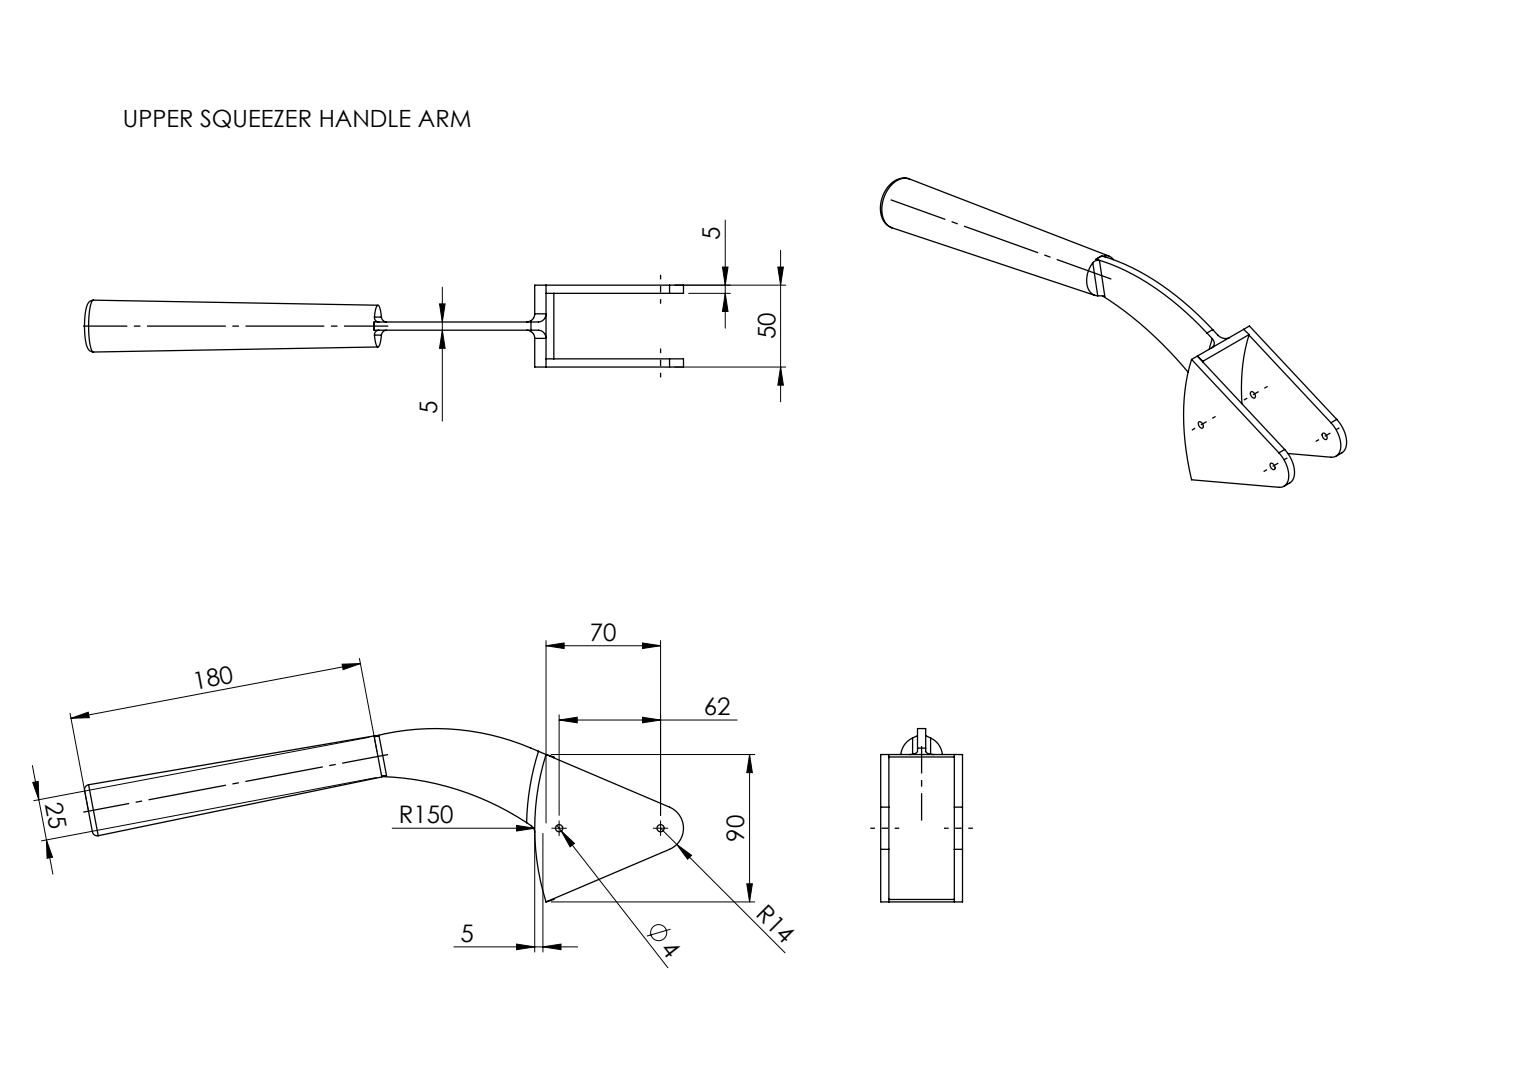
ISO-10303-21;
HEADER;
FILE_DESCRIPTION (('STEP AP214'),
    '1' );
FILE_NAME ('Upper Squeezer Handle Arm.step',
    '2026-10-02T13:02:33',
    ( '' ),
    ( '' ),
    'SwSTEP 2.0',
    'SolidWorks 2026',
    '' );
FILE_SCHEMA (( 'AUTOMOTIVE_DESIGN' ));
ENDSEC;

DATA;
#40=ORIENTED_EDGE ( 'NONE', *, *, #10473, .T. ) ;
#56=VERTEX_POINT ( 'NONE', #8559 ) ;
#88=DIRECTION ( 'NONE',  ( -0.000000000000000000, -0.000000000000000000, -1.000000000000000000 ) ) ;
#109=( NAMED_UNIT ( * ) SI_UNIT ( $, .STERADIAN. ) SOLID_ANGLE_UNIT ( ) );
#113=VERTEX_POINT ( 'NONE', #1359 ) ;
#130=FACE_OUTER_BOUND ( 'NONE', #4986, .T. ) ;
#141=DIRECTION ( 'NONE',  ( -1.000000000000000000, 0.000000000000000000, 0.000000000000000000 ) ) ;
#142=EDGE_LOOP ( 'NONE', ( #9264, #8766, #6960, #18741, #15276 ) ) ;
#165=CIRCLE ( 'NONE', #14403, 12.74754878398197633 ) ;
#196=CARTESIAN_POINT ( 'NONE',  ( -64.20000000000000284, 2.694222958124180951E-16, -25.00000000000000000 ) ) ;
#229=ORIENTED_EDGE ( 'NONE', *, *, #5595, .F. ) ;
#256=DIRECTION ( 'NONE',  ( 0.000000000000000000, 0.000000000000000000, 1.000000000000000000 ) ) ;
#276=ORIENTED_EDGE ( 'NONE', *, *, #13888, .T. ) ;
#288=DIRECTION ( 'NONE',  ( 0.9826218788918642533, 0.1856185419698762884, -0.000000000000000000 ) ) ;
#289=AXIS2_PLACEMENT_3D ( 'NONE', #791, #6676, #10995 ) ;
#326=ORIENTED_EDGE ( 'NONE', *, *, #13082, .F. ) ;
#359=EDGE_CURVE ( 'NONE', #9050, #9141, #4270, .T. ) ;
#361=DIRECTION ( 'NONE',  ( 0.000000000000000000, 0.000000000000000000, 1.000000000000000000 ) ) ;
#395=LINE ( 'NONE', #17952, #3848 ) ;
#411=VERTEX_POINT ( 'NONE', #18575 ) ;
#417=DIRECTION ( 'NONE',  ( 1.000000000000000000, 0.000000000000000000, 0.000000000000000000 ) ) ;
#426=TOROIDAL_SURFACE ( 'NONE', #13412, 155.0000000000000284, 5.000000000000000000 ) ;
#430=CARTESIAN_POINT ( 'NONE',  ( -349.0394899966146909, 23.59157312255261729, 2.567204941047426911E-15 ) ) ;
#468=LINE ( 'NONE', #1619, #12903 ) ;
#479=DIRECTION ( 'NONE',  ( -1.000000000000000000, 0.000000000000000000, 0.000000000000000000 ) ) ;
#496=CARTESIAN_POINT ( 'NONE',  ( -174.0670050711101737, 56.28339404658832024, -2.500000000000000000 ) ) ;
#512=CARTESIAN_POINT ( 'NONE',  ( 5.481473465377026066, -12.88229205725314586, -19.99999999999999645 ) ) ;
#518=VERTEX_POINT ( 'NONE', #6943 ) ;
#522=DIRECTION ( 'NONE',  ( -0.000000000000000000, -0.000000000000000000, -1.000000000000000000 ) ) ;
#530=FACE_BOUND ( 'NONE', #4136, .T. ) ;
#536=FACE_OUTER_BOUND ( 'NONE', #6098, .T. ) ;
#552=ADVANCED_FACE ( 'NONE', ( #6251 ), #11983, .T. ) ;
#558=LINE ( 'NONE', #16393, #11124 ) ;
#559=VECTOR ( 'NONE', #18084, 1000.000000000000000 ) ;
#563=FACE_OUTER_BOUND ( 'NONE', #9796, .T. ) ;
#564=EDGE_CURVE ( 'NONE', #10544, #13205, #12684, .T. ) ;
#574=CARTESIAN_POINT ( 'NONE',  ( -2.200000000000000178, 0.000000000000000000, 25.00000000000000000 ) ) ;
#575=CIRCLE ( 'NONE', #15701, 2.200000000000000622 ) ;
#607=VECTOR ( 'NONE', #8603, 1000.000000000000000 ) ;
#619=ORIENTED_EDGE ( 'NONE', *, *, #10277, .T. ) ;
#671=PLANE ( 'NONE',  #9426 ) ;
#679=CARTESIAN_POINT ( 'NONE',  ( -70.00000000000000000, 44.99999999999999289, -19.99999999999999645 ) ) ;
#718=CARTESIAN_POINT ( 'NONE',  ( -174.0586467429681363, 56.10169251196822415, -3.278196957010492962 ) ) ;
#742=DIRECTION ( 'NONE',  ( 0.000000000000000000, 0.000000000000000000, 1.000000000000000000 ) ) ;
#744=( LENGTH_UNIT ( ) NAMED_UNIT ( * ) SI_UNIT ( .MILLI., .METRE. ) );
#748=LINE ( 'NONE', #7752, #16988 ) ;
#751=DIRECTION ( 'NONE',  ( 1.000000000000000000, 0.000000000000000000, 0.000000000000000000 ) ) ;
#753=VERTEX_POINT ( 'NONE', #12822 ) ;
#780=CARTESIAN_POINT ( 'NONE',  ( 73.09088021254186174, 1.387778780781445676E-14, 25.00000000000000000 ) ) ;
#783=EDGE_CURVE ( 'NONE', #1828, #11020, #12691, .T. ) ;
#791=CARTESIAN_POINT ( 'NONE',  ( -70.00000000000000000, 44.99999999999999289, 2.500000000000000000 ) ) ;
#797=ORIENTED_EDGE ( 'NONE', *, *, #18408, .F. ) ;
#830=CIRCLE ( 'NONE', #16252, 2.200000000000007283 ) ;
#836=CARTESIAN_POINT ( 'NONE',  ( -346.6567719130321166, 10.97801148527007697, 9.951701414186830458E-16 ) ) ;
#844=DIRECTION ( 'NONE',  ( -0.000000000000000000, -0.000000000000000000, -1.000000000000000000 ) ) ;
#860=AXIS2_PLACEMENT_3D ( 'NONE', #11980, #10856, #3558 ) ;
#883=VECTOR ( 'NONE', #7257, 1000.000000000000000 ) ;
#897=VERTEX_POINT ( 'NONE', #15494 ) ;
#901=CARTESIAN_POINT ( 'NONE',  ( -168.2745196454702068, 32.00972194781247282, -2.584671478510871090 ) ) ;
#912=VECTOR ( 'NONE', #7964, 1000.000000000000000 ) ;
#918=CIRCLE ( 'NONE', #5451, 150.0000000000000284 ) ;
#955=EDGE_CURVE ( 'NONE', #4610, #5412, #8486, .T. ) ;
#985=EDGE_LOOP ( 'NONE', ( #11976, #13924 ) ) ;
#987=VECTOR ( 'NONE', #3572, 1000.000000000000000 ) ;
#997=CARTESIAN_POINT ( 'NONE',  ( 73.09088021254186174, 1.387778780781445676E-14, 7.500000000000000000 ) ) ;
#998=CARTESIAN_POINT ( 'NONE',  ( 73.09088021254186174, 1.387778780781445676E-14, -7.500000000000000000 ) ) ;
#1008=ORIENTED_EDGE ( 'NONE', *, *, #2884, .T. ) ;
#1058=CARTESIAN_POINT ( 'NONE',  ( 2.200000000000000178, 2.694222958124177006E-16, 25.00000000000000000 ) ) ;
#1064=CARTESIAN_POINT ( 'NONE',  ( -167.4745151998187680, 32.15905408292213252, 2.500000000000000000 ) ) ;
#1084=CARTESIAN_POINT ( 'NONE',  ( -170.4124675745486570, 31.54971992778986234, -5.500000000000000000 ) ) ;
#1099=CARTESIAN_POINT ( 'NONE',  ( -170.5500158571522320, 32.36820283781686669, 5.132104245558541500 ) ) ;
#1103=CARTESIAN_POINT ( 'NONE',  ( -70.00000000000000000, 44.99999999999999289, 7.500000000000007105 ) ) ;
#1128=CARTESIAN_POINT ( 'NONE',  ( 0.000000000000000000, 0.000000000000000000, 25.00000000000000000 ) ) ;
#1130=CARTESIAN_POINT ( 'NONE',  ( -65.23030399291528170, -43.49999999999991473, 19.99999999999993605 ) ) ;
#1144=ORIENTED_EDGE ( 'NONE', *, *, #12791, .F. ) ;
#1151=DIRECTION ( 'NONE',  ( -0.9826218788918642533, -0.1856185419698762884, 0.000000000000000000 ) ) ;
#1160=DIRECTION ( 'NONE',  ( 1.000000000000000000, 0.000000000000000000, 0.000000000000000000 ) ) ;
#1162=CIRCLE ( 'NONE', #11700, 145.0000000000000284 ) ;
#1165=DIRECTION ( 'NONE',  ( -0.000000000000000000, -0.000000000000000000, 1.000000000000000000 ) ) ;
#1181=LINE ( 'NONE', #16691, #8739 ) ;
#1194=FACE_OUTER_BOUND ( 'NONE', #3187, .T. ) ;
#1215=LINE ( 'NONE', #7000, #4553 ) ;
#1220=ADVANCED_FACE ( 'NONE', ( #9641 ), #2329, .T. ) ;
#1222=LINE ( 'NONE', #12750, #18237 ) ;
#1227=CIRCLE ( 'NONE', #16352, 12.74754878398197633 ) ;
#1235=CARTESIAN_POINT ( 'NONE',  ( -70.00000000000000000, 44.99999999999999289, 20.00000000000001776 ) ) ;
#1238=AXIS2_PLACEMENT_3D ( 'NONE', #16759, #16849, #17042 ) ;
#1258=ORIENTED_EDGE ( 'NONE', *, *, #6088, .F. ) ;
#1262=CARTESIAN_POINT ( 'NONE',  ( -170.4124675745486570, 31.54971992778987655, 2.500000000000000000 ) ) ;
#1280=CARTESIAN_POINT ( 'NONE',  ( -344.2740538294495423, -1.635550152012466452, 9.951701414186830458E-16 ) ) ;
#1299=CARTESIAN_POINT ( 'NONE',  ( -174.8673125818257006, 55.13264502119463373, 5.500000000000001776 ) ) ;
#1331=EDGE_CURVE ( 'NONE', #7954, #16292, #18686, .T. ) ;
#1337=CARTESIAN_POINT ( 'NONE',  ( 73.09088021254186174, 1.387778780781445676E-14, 19.99999999999997513 ) ) ;
#1339=DIRECTION ( 'NONE',  ( -0.3915338189555019333, 0.9201637183752250371, 0.000000000000000000 ) ) ;
#1344=PLANE ( 'NONE',  #13494 ) ;
#1359=CARTESIAN_POINT ( 'NONE',  ( -2.200000000000000178, 0.000000000000000000, -19.99999999999999645 ) ) ;
#1393=CARTESIAN_POINT ( 'NONE',  ( -175.0529311237955596, 56.11526690008648899, 2.500000000000000000 ) ) ;
#1405=FACE_OUTER_BOUND ( 'NONE', #1455, .T. ) ;
#1409=CARTESIAN_POINT ( 'NONE',  ( -170.4124675745486570, 31.54971992778987655, -2.500000000000000000 ) ) ;
#1410=ORIENTED_EDGE ( 'NONE', *, *, #11519, .F. ) ;
#1417=EDGE_CURVE ( 'NONE', #1906, #5889, #1222, .T. ) ;
#1455=EDGE_LOOP ( 'NONE', ( #13094, #13490 ) ) ;
#1475=CARTESIAN_POINT ( 'NONE',  ( -70.24339520416560845, 45.10356575889633746, -5.890567936347699707 ) ) ;
#1513=AXIS2_PLACEMENT_3D ( 'NONE', #9646, #10955, #3741 ) ;
#1515=DIRECTION ( 'NONE',  ( -2.671473304378624222E-16, -0.000000000000000000, -1.000000000000000000 ) ) ;
#1526=EDGE_LOOP ( 'NONE', ( #6897, #6518, #14749, #5534 ) ) ;
#1527=ADVANCED_FACE ( 'NONE', ( #13477 ), #6129, .T. ) ;
#1539=CARTESIAN_POINT ( 'NONE',  ( -76.95187462163347902, -1.796833398359349410, -6.747090334426651737 ) ) ;
#1549=DIRECTION ( 'NONE',  ( -0.000000000000000000, -0.000000000000000000, -1.000000000000000000 ) ) ;
#1566=AXIS2_PLACEMENT_3D ( 'NONE', #9927, #1151, #9845 ) ;
#1571=CARTESIAN_POINT ( 'NONE',  ( -76.90911978745816668, -45.00000000000000711, 20.00000000000002132 ) ) ;
#1600=ORIENTED_EDGE ( 'NONE', *, *, #16700, .T. ) ;
#1615=LINE ( 'NONE', #17277, #8663 ) ;
#1619=CARTESIAN_POINT ( 'NONE',  ( -69.99999999999998579, -45.00000000000000711, -19.99999999999999645 ) ) ;
#1624=ORIENTED_EDGE ( 'NONE', *, *, #11579, .F. ) ;
#1629=CARTESIAN_POINT ( 'NONE',  ( -77.83221577883584530, 0.3113175352389498385, -4.597871329320426526 ) ) ;
#1646=DIRECTION ( 'NONE',  ( -0.3000000000000013767, -0.9539392014169453260, 0.000000000000000000 ) ) ;
#1679=AXIS2_PLACEMENT_3D ( 'NONE', #1950, #4958, #16653 ) ;
#1681=CARTESIAN_POINT ( 'NONE',  ( 73.09088021254186174, 1.387778780781445676E-14, -2.500000000000000444 ) ) ;
#1706=AXIS2_PLACEMENT_3D ( 'NONE', #9851, #15620, #2647 ) ;
#1719=ORIENTED_EDGE ( 'NONE', *, *, #16557, .T. ) ;
#1720=ORIENTED_EDGE ( 'NONE', *, *, #1770, .F. ) ;
#1732=DIRECTION ( 'NONE',  ( -0.000000000000000000, -0.000000000000000000, 1.000000000000000000 ) ) ;
#1734=CARTESIAN_POINT ( 'NONE',  ( -70.46959788260221558, 45.19981602042874869, -5.279908564046689179 ) ) ;
#1770=EDGE_CURVE ( 'NONE', #11020, #1828, #4868, .T. ) ;
#1780=VECTOR ( 'NONE', #11064, 1000.000000000000114 ) ;
#1828=VERTEX_POINT ( 'NONE', #15612 ) ;
#1846=FACE_OUTER_BOUND ( 'NONE', #15073, .T. ) ;
#1855=AXIS2_PLACEMENT_3D ( 'NONE', #430, #3432, #1939 ) ;
#1863=DIRECTION ( 'NONE',  ( 0.000000000000000000, 0.000000000000000000, 1.000000000000000000 ) ) ;
#1883=ORIENTED_EDGE ( 'NONE', *, *, #14085, .T. ) ;
#1906=VERTEX_POINT ( 'NONE', #3176 ) ;
#1916=CARTESIAN_POINT ( 'NONE',  ( 5.481473465377021625, 12.88229205725314763, -19.99999999999998934 ) ) ;
#1923=DIRECTION ( 'NONE',  ( 0.9201637183752249260, -0.3915338189555017667, 0.000000000000000000 ) ) ;
#1936=DIRECTION ( 'NONE',  ( -0.000000000000000000, -0.000000000000000000, -1.000000000000000000 ) ) ;
#1939=DIRECTION ( 'NONE',  ( 0.000000000000000000, -1.000000000000000000, -1.203364738757079611E-16 ) ) ;
#1950=CARTESIAN_POINT ( 'NONE',  ( -76.90911978745816668, -45.00000000000000711, 20.00000000000002132 ) ) ;
#1980=ORIENTED_EDGE ( 'NONE', *, *, #10414, .F. ) ;
#1995=CARTESIAN_POINT ( 'NONE',  ( 73.09088021254186174, 1.387778780781445676E-14, 19.99999999999997513 ) ) ;
#2005=EDGE_CURVE ( 'NONE', #8575, #3590, #2409, .T. ) ;
#2012=PLANE ( 'NONE',  #13053 ) ;
#2027=DIRECTION ( 'NONE',  ( 0.000000000000000000, 0.000000000000000000, 1.000000000000000000 ) ) ;
#2035=CARTESIAN_POINT ( 'NONE',  ( -172.7326993491721225, 43.83249341393818810, 9.951701414186830458E-16 ) ) ;
#2068=DIRECTION ( 'NONE',  ( -0.3915338189555018222, -0.9201637183752250371, 0.000000000000000000 ) ) ;
#2073=CARTESIAN_POINT ( 'NONE',  ( -172.7326993491721225, 43.83249341393818810, 9.951701414186830458E-16 ) ) ;
#2082=CYLINDRICAL_SURFACE ( 'NONE', #10230, 13.99999999999999822 ) ;
#2097=ORIENTED_EDGE ( 'NONE', *, *, #3220, .T. ) ;
#2113=CARTESIAN_POINT ( 'NONE',  ( -73.13054148225640461, 46.33205954274173877, -2.756412765970647882 ) ) ;
#2121=AXIS2_PLACEMENT_3D ( 'NONE', #8067, #6961, #11086 ) ;
#2122=AXIS2_PLACEMENT_3D ( 'NONE', #10418, #12980, #8826 ) ;
#2124=CARTESIAN_POINT ( 'NONE',  ( -169.3344985746950044, 31.92300743893811088, 3.146712427857110583 ) ) ;
#2127=TOROIDAL_SURFACE ( 'NONE', #16361, 155.0000000000000284, 5.000000000000000000 ) ;
#2132=CARTESIAN_POINT ( 'NONE',  ( -175.0529311237955596, 56.11526690008648899, 2.500000000000000000 ) ) ;
#2138=VERTEX_POINT ( 'NONE', #7622 ) ;
#2144=VERTEX_POINT ( 'NONE', #4755 ) ;
#2147=CIRCLE ( 'NONE', #13934, 2.200000000000000178 ) ;
#2153=DIRECTION ( 'NONE',  ( 1.000000000000000000, 0.000000000000000000, -0.000000000000000000 ) ) ;
#2156=DIRECTION ( 'NONE',  ( -1.000000000000000000, 0.000000000000000000, 0.000000000000000000 ) ) ;
#2167=DIRECTION ( 'NONE',  ( 0.000000000000000000, 0.000000000000000000, 1.000000000000000000 ) ) ;
#2172=ADVANCED_FACE ( 'NONE', ( #10535 ), #2012, .F. ) ;
#2174=AXIS2_PLACEMENT_3D ( 'NONE', #12078, #3652, #16476 ) ;
#2196=FILL_AREA_STYLE ('',( #9865 ) ) ;
#2201=DIRECTION ( 'NONE',  ( -0.9201637183752250371, 0.3915338189555017667, 2.458192809297184296E-16 ) ) ;
#2209=EDGE_CURVE ( 'NONE', #4027, #10083, #12700, .T. ) ;
#2212=ORIENTED_EDGE ( 'NONE', *, *, #9806, .T. ) ;
#2231=ORIENTED_EDGE ( 'NONE', *, *, #18528, .T. ) ;
#2232=CARTESIAN_POINT ( 'NONE',  ( -79.20163718375225415, 48.91533818955501545, 2.500000000000000000 ) ) ;
#2260=CARTESIAN_POINT ( 'NONE',  ( -80.88842949533930948, 2.743677230443736903, -2.574918967431987227 ) ) ;
#2268=DIRECTION ( 'NONE',  ( -0.9826218788918642533, -0.1856185419698762884, 0.000000000000000000 ) ) ;
#2276=FACE_BOUND ( 'NONE', #7402, .T. ) ;
#2285=FACE_OUTER_BOUND ( 'NONE', #5660, .T. ) ;
#2290=LINE ( 'NONE', #8071, #9863 ) ;
#2295=CARTESIAN_POINT ( 'NONE',  ( -169.9074338689577530, 31.96868808717145782, -3.724467847532850762 ) ) ;
#2305=CARTESIAN_POINT ( 'NONE',  ( -74.62210677719829732, 46.96672731380024146, 2.500000000000000000 ) ) ;
#2315=ORIENTED_EDGE ( 'NONE', *, *, #14957, .T. ) ;
#2329=PLANE ( 'NONE',  #12706 ) ;
#2359=CARTESIAN_POINT ( 'NONE',  ( -69.99999999999998579, -45.00000000000000711, 25.00000000000000000 ) ) ;
#2372=EDGE_CURVE ( 'NONE', #14394, #2138, #11538, .T. ) ;
#2389=CARTESIAN_POINT ( 'NONE',  ( -170.5980861165185445, 32.53234180668174247, -5.500000000000001776 ) ) ;
#2397=ORIENTED_EDGE ( 'NONE', *, *, #5880, .F. ) ;
#2408=CARTESIAN_POINT ( 'NONE',  ( -72.99658078354744362, 46.27505866028131010, 2.816616659167352044 ) ) ;
#2409=LINE ( 'NONE', #11012, #5208 ) ;
#2415=ORIENTED_EDGE ( 'NONE', *, *, #16291, .F. ) ;
#2441=DIRECTION ( 'NONE',  ( 0.1856185419698762884, -0.9826218788918642533, 0.000000000000000000 ) ) ;
#2446=DIRECTION ( 'NONE',  ( 0.000000000000000000, 0.000000000000000000, 1.000000000000000000 ) ) ;
#2453=LINE ( 'NONE', #1058, #9909 ) ;
#2465=CARTESIAN_POINT ( 'NONE',  ( -79.48103206242137730, 1.792378103397237687, -3.092380961970916609 ) ) ;
#2472=AXIS2_PLACEMENT_3D ( 'NONE', #5439, #3997, #13856 ) ;
#2481=FACE_BOUND ( 'NONE', #6430, .T. ) ;
#2508=CARTESIAN_POINT ( 'NONE',  ( -71.81027153490798298, 45.77027871590120611, 3.518396351564663682 ) ) ;
#2530=CARTESIAN_POINT ( 'NONE',  ( -167.4745151998187680, 32.15905408292206147, -2.500000000000000000 ) ) ;
#2557=CYLINDRICAL_SURFACE ( 'NONE', #16277, 2.200000000000000622 ) ;
#2572=ORIENTED_EDGE ( 'NONE', *, *, #16811, .F. ) ;
#2574=ADVANCED_FACE ( 'NONE', ( #8157 ), #8849, .T. ) ;
#2575=ORIENTED_EDGE ( 'NONE', *, *, #4514, .T. ) ;
#2594=VECTOR ( 'NONE', #13746, 1000.000000000000000 ) ;
#2595=CARTESIAN_POINT ( 'NONE',  ( -70.03008040050728766, 45.01279934630233015, 6.841710791646147705 ) ) ;
#2597=CARTESIAN_POINT ( 'NONE',  ( 0.000000000000000000, 0.000000000000000000, -19.99999999999999645 ) ) ;
#2626=CARTESIAN_POINT ( 'NONE',  ( -76.94165664733894516, -1.794943808410583763, 6.745229976240270098 ) ) ;
#2647=DIRECTION ( 'NONE',  ( -1.000000000000000000, 0.000000000000000000, 0.000000000000000000 ) ) ;
#2660=EDGE_CURVE ( 'NONE', #18388, #3138, #17169, .T. ) ;
#2664=AXIS2_PLACEMENT_3D ( 'NONE', #4048, #15343, #8340 ) ;
#2687=ADVANCED_FACE ( 'NONE', ( #15728 ), #2557, .F. ) ;
#2691=ADVANCED_FACE ( 'NONE', ( #17279, #6940, #5509 ), #1344, .F. ) ;
#2731=B_SPLINE_CURVE_WITH_KNOTS ( 'NONE', 3,
 ( #15742, #17379, #4363, #12879 ),
 .UNSPECIFIED., .F., .F.,
 ( 4, 4 ),
 ( 0.000000000000000000, 0.003000475340473851647 ),
 .UNSPECIFIED. ) ;
#2740=CARTESIAN_POINT ( 'NONE',  ( -168.4538323585589694, 31.95594125380575434, 2.500000000000000000 ) ) ;
#2744=PLANE ( 'NONE',  #4472 ) ;
#2764=EDGE_LOOP ( 'NONE', ( #5604, #4078, #18302, #15584 ) ) ;
#2770=CARTESIAN_POINT ( 'NONE',  ( -77.50987606495345972, -0.1965428547086033040, -5.115516238835398966 ) ) ;
#2787=B_SPLINE_CURVE_WITH_KNOTS ( 'NONE', 3,
 ( #2389, #15281, #16923, #13956, #12524, #10912, #15377, #2295, #6578, #18367, #12327, #13849, #16736, #901, #12436, #5340 ),
 .UNSPECIFIED., .F., .F.,
 ( 4, 2, 2, 2, 2, 2, 2, 4 ),
 ( 1.734723475976807094E-18, 0.0006035471611761681829, 0.001207094322352334631, 0.001810641483528501296, 0.002414188644704666660, 0.003017735805880831807, 0.003621282967056997388, 0.004828377289409254390 ),
 .UNSPECIFIED. ) ;
#2827=ORIENTED_EDGE ( 'NONE', *, *, #2372, .T. ) ;
#2853=DIRECTION ( 'NONE',  ( -0.1856185419698762884, 0.9826218788918642533, 0.000000000000000000 ) ) ;
#2859=DIRECTION ( 'NONE',  ( 1.000000000000000000, 0.000000000000000000, 0.000000000000000000 ) ) ;
#2868=CARTESIAN_POINT ( 'NONE',  ( -172.8945038000772456, 56.46685571404672999, 2.584671478510881748 ) ) ;
#2872=CARTESIAN_POINT ( 'NONE',  ( -70.03007184274690644, 45.01279570493660742, -6.843761338458851817 ) ) ;
#2884=EDGE_CURVE ( 'NONE', #12460, #518, #18423, .T. ) ;
#2899=ORIENTED_EDGE ( 'NONE', *, *, #11873, .T. ) ;
#2903=EDGE_CURVE ( 'NONE', #14167, #1906, #558, .T. ) ;
#2923=ORIENTED_EDGE ( 'NONE', *, *, #17865, .F. ) ;
#2927=CIRCLE ( 'NONE', #13510, 155.0000000000000284 ) ;
#2931=DIRECTION ( 'NONE',  ( 1.000000000000000000, 0.000000000000000000, -0.000000000000000000 ) ) ;
#2954=EDGE_LOOP ( 'NONE', ( #14575, #6574, #14958, #16245 ) ) ;
#2964=ORIENTED_EDGE ( 'NONE', *, *, #17775, .T. ) ;
#2966=CARTESIAN_POINT ( 'NONE',  ( 0.000000000000000000, 0.000000000000000000, 25.00000000000000000 ) ) ;
#2970=AXIS2_PLACEMENT_3D ( 'NONE', #2966, #4104, #141 ) ;
#2986=PLANE ( 'NONE',  #12549 ) ;
#3010=LINE ( 'NONE', #12955, #8538 ) ;
#3012=DIRECTION ( 'NONE',  ( 1.000000000000000000, 0.000000000000000000, 0.000000000000000000 ) ) ;
#3014=CARTESIAN_POINT ( 'NONE',  ( 0.000000000000000000, 0.000000000000000000, 20.00000000000000000 ) ) ;
#3037=CIRCLE ( 'NONE', #9719, 171.3327290851023292 ) ;
#3062=EDGE_LOOP ( 'NONE', ( #8219, #13627 ) ) ;
#3066=CARTESIAN_POINT ( 'NONE',  ( -174.8824303167912717, 55.30300876447670788, -5.132104245558540612 ) ) ;
#3067=CARTESIAN_POINT ( 'NONE',  ( -71.14323843904776368, 45.48645312032893173, -4.192014029982320977 ) ) ;
#3069=ORIENTED_EDGE ( 'NONE', *, *, #16811, .T. ) ;
#3083=DIRECTION ( 'NONE',  ( -0.000000000000000000, -0.000000000000000000, -1.000000000000000000 ) ) ;
#3087=ORIENTED_EDGE ( 'NONE', *, *, #4173, .F. ) ;
#3123=EDGE_CURVE ( 'NONE', #753, #7914, #8693, .T. ) ;
#3138=VERTEX_POINT ( 'NONE', #17523 ) ;
#3147=DIRECTION ( 'NONE',  ( 1.000000000000000000, 0.000000000000000000, 0.000000000000000000 ) ) ;
#3148=DIRECTION ( 'NONE',  ( 0.9201637183752249260, 0.3915338189555018777, -2.458192809297183803E-16 ) ) ;
#3176=CARTESIAN_POINT ( 'NONE',  ( -69.99999999999998579, -45.00000000000000711, 20.00000000000001776 ) ) ;
#3187=EDGE_LOOP ( 'NONE', ( #7835, #12831, #11103, #4991, #2315, #2899 ) ) ;
#3197=DIRECTION ( 'NONE',  ( 0.1856185419698760941, -0.9826218788918640312, 0.000000000000000000 ) ) ;
#3204=ORIENTED_EDGE ( 'NONE', *, *, #4750, .F. ) ;
#3209=ORIENTED_EDGE ( 'NONE', *, *, #18358, .F. ) ;
#3220=EDGE_CURVE ( 'NONE', #12815, #17451, #5025, .T. ) ;
#3230=VERTEX_POINT ( 'NONE', #15890 ) ;
#3249=DIRECTION ( 'NONE',  ( 1.000000000000000000, 0.000000000000000000, -2.671473304378624222E-16 ) ) ;
#3284=ORIENTED_EDGE ( 'NONE', *, *, #4389, .T. ) ;
#3293=VECTOR ( 'NONE', #7540, 1000.000000000000000 ) ;
#3295=CARTESIAN_POINT ( 'NONE',  ( -76.88766983611584749, -2.536636612185957595, -7.500000000000000000 ) ) ;
#3309=DIRECTION ( 'NONE',  ( 0.9201637183752249260, 0.3915338189555018777, 0.000000000000000000 ) ) ;
#3314=CARTESIAN_POINT ( 'NONE',  ( -59.79999999999999716, 0.000000000000000000, -25.00000000000000000 ) ) ;
#3326=CARTESIAN_POINT ( 'NONE',  ( -70.00000000000000000, 44.99999999999999289, 25.00000000000000000 ) ) ;
#3332=FACE_OUTER_BOUND ( 'NONE', #1526, .T. ) ;
#3362=ORIENTED_EDGE ( 'NONE', *, *, #18484, .T. ) ;
#3390=PRODUCT_DEFINITION_CONTEXT ( 'detailed design', #12682, 'design' ) ;
#3400=DIRECTION ( 'NONE',  ( -0.000000000000000000, -0.000000000000000000, -1.000000000000000000 ) ) ;
#3413=TOROIDAL_SURFACE ( 'NONE', #5868, 12.83663829214476770, 3.000000000000000000 ) ;
#3429=DIRECTION ( 'NONE',  ( -0.9826218788918641422, -0.1856185419698762606, 0.000000000000000000 ) ) ;
#3432=DIRECTION ( 'NONE',  ( 2.273171532858076093E-17, -1.203364738757079611E-16, 1.000000000000000000 ) ) ;
#3438=DIRECTION ( 'NONE',  ( -0.9826218788918642533, -0.1856185419698762884, 0.000000000000000000 ) ) ;
#3439=CARTESIAN_POINT ( 'NONE',  ( 73.09088021254186174, 1.387778780781445676E-14, -19.99999999999999645 ) ) ;
#3456=CYLINDRICAL_SURFACE ( 'NONE', #10978, 150.0000000000000284 ) ;
#3457=CARTESIAN_POINT ( 'NONE',  ( -172.7326993491721225, 43.83249341393818810, 9.951701414186830458E-16 ) ) ;
#3492=ORIENTED_EDGE ( 'NONE', *, *, #7729, .F. ) ;
#3496=ORIENTED_EDGE ( 'NONE', *, *, #6088, .T. ) ;
#3513=DIRECTION ( 'NONE',  ( 0.000000000000000000, 0.000000000000000000, 1.000000000000000000 ) ) ;
#3517=ORIENTED_EDGE ( 'NONE', *, *, #8216, .T. ) ;
#3530=DIRECTION ( 'NONE',  ( -0.000000000000000000, -0.000000000000000000, -1.000000000000000000 ) ) ;
#3537=ORIENTED_EDGE ( 'NONE', *, *, #18192, .T. ) ;
#3543=EDGE_LOOP ( 'NONE', ( #7602, #3069 ) ) ;
#3558=DIRECTION ( 'NONE',  ( 1.000000000000000000, 0.000000000000000000, 0.000000000000000000 ) ) ;
#3561=EDGE_CURVE ( 'NONE', #10291, #16721, #11039, .T. ) ;
#3572=DIRECTION ( 'NONE',  ( -0.000000000000000000, -0.000000000000000000, -1.000000000000000000 ) ) ;
#3573=UNCERTAINTY_MEASURE_WITH_UNIT (LENGTH_MEASURE( 1.000000000000000082E-05 ), #744, 'distance_accuracy_value', 'NONE');
#3581=EDGE_CURVE ( 'NONE', #16919, #13271, #5387, .T. ) ;
#3590=VERTEX_POINT ( 'NONE', #1235 ) ;
#3593=CARTESIAN_POINT ( 'NONE',  ( 2.200000000000000178, 2.694222958124177006E-16, -25.00000000000000000 ) ) ;
#3614=LINE ( 'NONE', #12527, #11561 ) ;
#3622=LINE ( 'NONE', #9430, #3293 ) ;
#3637=ORIENTED_EDGE ( 'NONE', *, *, #4750, .T. ) ;
#3644=ORIENTED_EDGE ( 'NONE', *, *, #3220, .F. ) ;
#3652=DIRECTION ( 'NONE',  ( 0.000000000000000000, 0.000000000000000000, 1.000000000000000000 ) ) ;
#3662=AXIS2_PLACEMENT_3D ( 'NONE', #12821, #5908, #17400 ) ;
#3663=CARTESIAN_POINT ( 'NONE',  ( -69.99999999999998579, -45.00000000000000711, 25.00000000000000000 ) ) ;
#3669=DIRECTION ( 'NONE',  ( -0.9826218788918641422, -0.1856185419698762606, 0.000000000000000000 ) ) ;
#3674=DIRECTION ( 'NONE',  ( -0.3915338189555019333, 0.9201637183752250371, 0.000000000000000000 ) ) ;
#3687=ORIENTED_EDGE ( 'NONE', *, *, #4439, .F. ) ;
#3690=PLANE ( 'NONE',  #13481 ) ;
#3695=ORIENTED_EDGE ( 'NONE', *, *, #7288, .F. ) ;
#3697=AXIS2_PLACEMENT_3D ( 'NONE', #8454, #13163, #2931 ) ;
#3702=DIRECTION ( 'NONE',  ( 1.000000000000000000, 0.000000000000000000, 0.000000000000000000 ) ) ;
#3705=VERTEX_POINT ( 'NONE', #9314 ) ;
#3707=DIRECTION ( 'NONE',  ( 3.816390434826605238E-17, 0.000000000000000000, -1.000000000000000000 ) ) ;
#3741=DIRECTION ( 'NONE',  ( 1.000000000000000000, 0.000000000000000000, 0.000000000000000000 ) ) ;
#3757=ORIENTED_EDGE ( 'NONE', *, *, #4389, .F. ) ;
#3758=CARTESIAN_POINT ( 'NONE',  ( -2.200000000000000178, 0.000000000000000000, -25.00000000000000000 ) ) ;
#3775=VERTEX_POINT ( 'NONE', #14690 ) ;
#3787=EDGE_CURVE ( 'NONE', #4836, #16919, #17591, .T. ) ;
#3842=ORIENTED_EDGE ( 'NONE', *, *, #1417, .F. ) ;
#3843=CARTESIAN_POINT ( 'NONE',  ( -170.3665179301995352, 31.30647307655612366, 9.951701414186830458E-16 ) ) ;
#3846=EDGE_LOOP ( 'NONE', ( #11783, #18763 ) ) ;
#3848=VECTOR ( 'NONE', #9283, 1000.000000000000000 ) ;
#3861=COLOUR_RGB ( '', 0.08235294, 0.09019608, 0.10196078) ;
#3868=CIRCLE ( 'NONE', #14792, 155.0000000000000284 ) ;
#3878=DIRECTION ( 'NONE',  ( 1.000000000000000000, 0.000000000000000000, 0.000000000000000000 ) ) ;
#3879=DIRECTION ( 'NONE',  ( -0.000000000000000000, -0.000000000000000000, -1.000000000000000000 ) ) ;
#3892=CARTESIAN_POINT ( 'NONE',  ( -170.3886569253285188, 32.16932146890094657, 4.579216830445319353 ) ) ;
#3900=CARTESIAN_POINT ( 'NONE',  ( -73.43026588874043625, 46.45959363168854139, 2.666351014094141547 ) ) ;
#3913=ORIENTED_EDGE ( 'NONE', *, *, #1417, .T. ) ;
#3930=DIRECTION ( 'NONE',  ( -0.9201637183752248150, 0.3915338189555022108, 0.000000000000000000 ) ) ;
#3933=CARTESIAN_POINT ( 'NONE',  ( -136.4286012789710867, -132.1908753210555574, 5.500000000000000000 ) ) ;
#3946=FACE_OUTER_BOUND ( 'NONE', #12937, .T. ) ;
#3956=CARTESIAN_POINT ( 'NONE',  ( -76.90911978745816668, 1.387778780781445676E-14, -25.00000000000000000 ) ) ;
#3959=CARTESIAN_POINT ( 'NONE',  ( 73.09088021254186174, 1.387778780781445676E-14, -19.99999999999999645 ) ) ;
#3963=AXIS2_PLACEMENT_3D ( 'NONE', #14828, #522, #11945 ) ;
#3988=ADVANCED_FACE ( 'NONE', ( #3946 ), #5492, .F. ) ;
#3991=ORIENTED_EDGE ( 'NONE', *, *, #955, .T. ) ;
#3995=ORIENTED_EDGE ( 'NONE', *, *, #15798, .F. ) ;
#3997=DIRECTION ( 'NONE',  ( -0.000000000000000000, -0.000000000000000000, -1.000000000000000000 ) ) ;
#4024=DIRECTION ( 'NONE',  ( -0.000000000000000000, -0.000000000000000000, -1.000000000000000000 ) ) ;
#4027=VERTEX_POINT ( 'NONE', #15006 ) ;
#4029=DIRECTION ( 'NONE',  ( 1.000000000000000000, 0.000000000000000000, 0.000000000000000000 ) ) ;
#4045=ORIENTED_EDGE ( 'NONE', *, *, #2005, .T. ) ;
#4048=CARTESIAN_POINT ( 'NONE',  ( -346.6053245638183853, 10.98772995598034008, 9.951701414186830458E-16 ) ) ;
#4052=DIRECTION ( 'NONE',  ( -0.000000000000000000, -0.000000000000000000, 1.000000000000000000 ) ) ;
#4078=ORIENTED_EDGE ( 'NONE', *, *, #17715, .F. ) ;
#4104=DIRECTION ( 'NONE',  ( -0.000000000000000000, -0.000000000000000000, -1.000000000000000000 ) ) ;
#4111=ORIENTED_EDGE ( 'NONE', *, *, #15798, .T. ) ;
#4128=CARTESIAN_POINT ( 'NONE',  ( -77.95464380949736949, 0.4739080578470992178, 4.432241562448437477 ) ) ;
#4131=AXIS2_PLACEMENT_3D ( 'NONE', #11782, #7456, #15981 ) ;
#4136=EDGE_LOOP ( 'NONE', ( #8783, #11844 ) ) ;
#4139=AXIS2_PLACEMENT_3D ( 'NONE', #6629, #2167, #13706 ) ;
#4167=FACE_OUTER_BOUND ( 'NONE', #11262, .T. ) ;
#4168=PRODUCT_DEFINITION_FORMATION_WITH_SPECIFIED_SOURCE ( 'ANY', '', #18543, .NOT_KNOWN. ) ;
#4170=DIRECTION ( 'NONE',  ( -0.000000000000000000, -0.000000000000000000, -1.000000000000000000 ) ) ;
#4173=EDGE_CURVE ( 'NONE', #5191, #11722, #3037, .T. ) ;
#4205=FACE_BOUND ( 'NONE', #985, .T. ) ;
#4215=EDGE_LOOP ( 'NONE', ( #13219, #12560, #3284, #14554, #6804, #15849 ) ) ;
#4216=LINE ( 'NONE', #1393, #13033 ) ;
#4235=CARTESIAN_POINT ( 'NONE',  ( -76.88766983611584749, -2.536636612185957595, 7.500000000000000000 ) ) ;
#4243=CIRCLE ( 'NONE', #7576, 13.99999999999999822 ) ;
#4255=LINE ( 'NONE', #8540, #1780 ) ;
#4266=EDGE_CURVE ( 'NONE', #12815, #15547, #1215, .T. ) ;
#4270=B_SPLINE_CURVE_WITH_KNOTS ( 'NONE', 3,
 ( #16744, #13757, #9518, #13857, #13964, #12529, #14053, #2124, #16635, #18285, #7912, #13672, #18374, #3892, #9722, #1099, #4385, #18664 ),
 .UNSPECIFIED., .F., .F.,
 ( 4, 2, 2, 2, 2, 2, 2, 2, 4 ),
 ( 1.734723475976807094E-18, 0.0006036110467294001801, 0.001207222093458798625, 0.001810833140188197179, 0.002414444186917595516, 0.003018055233646994937, 0.003621666280376394792, 0.004225277327105794213, 0.004828888373835193634 ),
 .UNSPECIFIED. ) ;
#4308=CARTESIAN_POINT ( 'NONE',  ( -70.00000000000001421, 44.99999999999998579, -7.500000000000000000 ) ) ;
#4328=CARTESIAN_POINT ( 'NONE',  ( -65.23030399291525327, 43.49999999999997868, -19.99999999999999645 ) ) ;
#4333=VERTEX_POINT ( 'NONE', #3758 ) ;
#4338=AXIS2_PLACEMENT_3D ( 'NONE', #3933, #2441, #7841 ) ;
#4363=CARTESIAN_POINT ( 'NONE',  ( -173.0810787726268245, 56.45151975169577696, 2.500000000000000000 ) ) ;
#4385=CARTESIAN_POINT ( 'NONE',  ( -170.5817629592740730, 32.44593076567889511, 5.316127001577102718 ) ) ;
#4389=EDGE_CURVE ( 'NONE', #6775, #16721, #15902, .T. ) ;
#4390=CARTESIAN_POINT ( 'NONE',  ( -174.8056419950568738, 55.54559466234915277, 4.582591203971079885 ) ) ;
#4397=ORIENTED_EDGE ( 'NONE', *, *, #564, .F. ) ;
#4403=VERTEX_POINT ( 'NONE', #8124 ) ;
#4405=AXIS2_PLACEMENT_3D ( 'NONE', #1571, #17325, #16154 ) ;
#4421=VECTOR ( 'NONE', #5232, 1000.000000000000000 ) ;
#4439=EDGE_CURVE ( 'NONE', #18049, #5889, #4596, .T. ) ;
#4451=ORIENTED_EDGE ( 'NONE', *, *, #2660, .T. ) ;
#4466=EDGE_LOOP ( 'NONE', ( #4740, #8137, #4584, #3204 ) ) ;
#4472=AXIS2_PLACEMENT_3D ( 'NONE', #5791, #1339, #11705 ) ;
#4474=EDGE_CURVE ( 'NONE', #6623, #4333, #15770, .T. ) ;
#4482=CARTESIAN_POINT ( 'NONE',  ( -174.6915139316591024, 55.69864286368945017, 4.224609204322596234 ) ) ;
#4484=( GEOMETRIC_REPRESENTATION_CONTEXT ( 3 ) GLOBAL_UNCERTAINTY_ASSIGNED_CONTEXT ( ( #3573 ) ) GLOBAL_UNIT_ASSIGNED_CONTEXT ( ( #744, #5284, #18405 ) ) REPRESENTATION_CONTEXT ( 'NONE', 'WORKASPACE' ) );
#4486=CARTESIAN_POINT ( 'NONE',  ( -174.8047394602870384, 55.54704694713838364, -4.579216830445309583 ) ) ;
#4492=ORIENTED_EDGE ( 'NONE', *, *, #5044, .F. ) ;
#4494=CIRCLE ( 'NONE', #17835, 149.4844750268701148 ) ;
#4500=DIRECTION ( 'NONE',  ( 0.000000000000000000, 0.000000000000000000, 1.000000000000000000 ) ) ;
#4509=CARTESIAN_POINT ( 'NONE',  ( 0.000000000000000000, 0.000000000000000000, 20.00000000000000000 ) ) ;
#4514=EDGE_CURVE ( 'NONE', #3138, #6411, #10096, .T. ) ;
#4515=ADVANCED_FACE ( 'NONE', ( #12928 ), #10370, .F. ) ;
#4538=VECTOR ( 'NONE', #2201, 1000.000000000000000 ) ;
#4539=VERTEX_POINT ( 'NONE', #17338 ) ;
#4553=VECTOR ( 'NONE', #5561, 1000.000000000000000 ) ;
#4567=CARTESIAN_POINT ( 'NONE',  ( -172.0951522251743029, 56.61964399677355431, -2.500000000000000000 ) ) ;
#4582=CARTESIAN_POINT ( 'NONE',  ( -72.57555729771728181, 46.09591126511114112, -3.005167547231827996 ) ) ;
#4584=ORIENTED_EDGE ( 'NONE', *, *, #783, .F. ) ;
#4587=CARTESIAN_POINT ( 'NONE',  ( 0.000000000000000000, 0.000000000000000000, 25.00000000000000000 ) ) ;
#4593=CIRCLE ( 'NONE', #13675, 12.74754878398197633 ) ;
#4596=LINE ( 'NONE', #10281, #14847 ) ;
#4607=EDGE_CURVE ( 'NONE', #10635, #897, #9327, .T. ) ;
#4610=VERTEX_POINT ( 'NONE', #18079 ) ;
#4626=EDGE_CURVE ( 'NONE', #7186, #3590, #3622, .T. ) ;
#4634=ORIENTED_EDGE ( 'NONE', *, *, #4607, .F. ) ;
#4635=ORIENTED_EDGE ( 'NONE', *, *, #11579, .T. ) ;
#4678=DIRECTION ( 'NONE',  ( 2.671473304378624222E-16, 0.000000000000000000, 1.000000000000000000 ) ) ;
#4686=ORIENTED_EDGE ( 'NONE', *, *, #6296, .T. ) ;
#4691=ORIENTED_EDGE ( 'NONE', *, *, #6028, .F. ) ;
#4700=FACE_OUTER_BOUND ( 'NONE', #4466, .T. ) ;
#4702=CARTESIAN_POINT ( 'NONE',  ( 0.000000000000000000, 0.000000000000000000, -19.99999999999999645 ) ) ;
#4723=EDGE_CURVE ( 'NONE', #16662, #15554, #8642, .T. ) ;
#4724=CARTESIAN_POINT ( 'NONE',  ( -76.88921716020503538, -2.445151130096096193, -7.406988961241581571 ) ) ;
#4740=ORIENTED_EDGE ( 'NONE', *, *, #18528, .F. ) ;
#4750=EDGE_CURVE ( 'NONE', #3775, #1828, #16035, .T. ) ;
#4753=VECTOR ( 'NONE', #9266, 1000.000000000000000 ) ;
#4755=CARTESIAN_POINT ( 'NONE',  ( -175.0529311237955881, 56.11526690008648899, -2.500000000000065725 ) ) ;
#4768=DIRECTION ( 'NONE',  ( 0.1856185419698762329, -0.9826218788918640312, 0.000000000000000000 ) ) ;
#4788=ORIENTED_EDGE ( 'NONE', *, *, #10414, .T. ) ;
#4797=DIRECTION ( 'NONE',  ( -0.9826218788918642533, -0.1856185419698762884, 0.000000000000000000 ) ) ;
#4802=DIRECTION ( 'NONE',  ( 0.000000000000000000, 0.000000000000000000, 1.000000000000000000 ) ) ;
#4811=ADVANCED_FACE ( 'NONE', ( #12811 ), #8650, .F. ) ;
#4833=CARTESIAN_POINT ( 'NONE',  ( -172.0951522251743029, 56.61964399677356141, 2.500000000000000000 ) ) ;
#4834=ORIENTED_EDGE ( 'NONE', *, *, #17615, .F. ) ;
#4836=VERTEX_POINT ( 'NONE', #8835 ) ;
#4845=CARTESIAN_POINT ( 'NONE',  ( -76.90911978745816668, 1.387778780781445676E-14, 25.00000000000000000 ) ) ;
#4864=CIRCLE ( 'NONE', #14259, 2.200000000000000622 ) ;
#4868=CIRCLE ( 'NONE', #1566, 12.83663829214476948 ) ;
#4907=ORIENTED_EDGE ( 'NONE', *, *, #6638, .T. ) ;
#4934=FACE_OUTER_BOUND ( 'NONE', #6975, .T. ) ;
#4936=DIRECTION ( 'NONE',  ( -1.000000000000000000, 0.000000000000000000, 0.000000000000000000 ) ) ;
#4941=CARTESIAN_POINT ( 'NONE',  ( 73.09088021254186174, 1.387778780781445676E-14, -19.99999999999999645 ) ) ;
#4943=ORIENTED_EDGE ( 'NONE', *, *, #8216, .F. ) ;
#4944=DIRECTION ( 'NONE',  ( 0.000000000000000000, 0.000000000000000000, 1.000000000000000000 ) ) ;
#4950=EDGE_CURVE ( 'NONE', #1906, #10635, #6165, .T. ) ;
#4954=ORIENTED_EDGE ( 'NONE', *, *, #3581, .T. ) ;
#4958=DIRECTION ( 'NONE',  ( 2.671473304378624222E-16, 0.000000000000000000, 1.000000000000000000 ) ) ;
#4959=ORIENTED_EDGE ( 'NONE', *, *, #15456, .T. ) ;
#4986=EDGE_LOOP ( 'NONE', ( #7336, #619, #17971, #18122, #2397, #3995 ) ) ;
#4991=ORIENTED_EDGE ( 'NONE', *, *, #4607, .T. ) ;
#5008=AXIS2_PLACEMENT_3D ( 'NONE', #3014, #8626, #5878 ) ;
#5025=CIRCLE ( 'NONE', #4131, 13.99999999999999822 ) ;
#5028=CIRCLE ( 'NONE', #10773, 12.74754878398197633 ) ;
#5044=EDGE_CURVE ( 'NONE', #17089, #9050, #11146, .T. ) ;
#5055=CARTESIAN_POINT ( 'NONE',  ( -64.20000000000000284, 2.694222958124175527E-16, 25.00000000000000000 ) ) ;
#5060=DIRECTION ( 'NONE',  ( 1.000000000000000000, 0.000000000000000000, 0.000000000000000000 ) ) ;
#5074=SURFACE_STYLE_USAGE ( .BOTH. , #13996 ) ;
#5077=VECTOR ( 'NONE', #6211, 999.9999999999998863 ) ;
#5082=CARTESIAN_POINT ( 'NONE',  ( 73.09088021254186174, 1.387778780781445676E-14, -7.500000000000000000 ) ) ;
#5092=ORIENTED_EDGE ( 'NONE', *, *, #17409, .F. ) ;
#5101=CIRCLE ( 'NONE', #7834, 12.74754878398197633 ) ;
#5117=VECTOR ( 'NONE', #14676, 1000.000000000000227 ) ;
#5120=ORIENTED_EDGE ( 'NONE', *, *, #13738, .F. ) ;
#5134=ORIENTED_EDGE ( 'NONE', *, *, #12741, .T. ) ;
#5143=DIRECTION ( 'NONE',  ( 1.000000000000000000, 0.000000000000000000, 0.000000000000000000 ) ) ;
#5165=CARTESIAN_POINT ( 'NONE',  ( -70.15002351626573329, 45.06383568389368577, 6.194099995621382249 ) ) ;
#5176=ORIENTED_EDGE ( 'NONE', *, *, #8295, .T. ) ;
#5191=VERTEX_POINT ( 'NONE', #1409 ) ;
#5208=VECTOR ( 'NONE', #11210, 1000.000000000000000 ) ;
#5232=DIRECTION ( 'NONE',  ( -0.000000000000000000, -0.000000000000000000, -1.000000000000000000 ) ) ;
#5244=LINE ( 'NONE', #18273, #2594 ) ;
#5284=( NAMED_UNIT ( * ) PLANE_ANGLE_UNIT ( ) SI_UNIT ( $, .RADIAN. ) );
#5291=CARTESIAN_POINT ( 'NONE',  ( -76.89394439365321432, -2.165653619537352803, 7.122830718932430472 ) ) ;
#5318=EDGE_CURVE ( 'NONE', #2138, #18388, #9390, .T. ) ;
#5324=ADVANCED_FACE ( 'NONE', ( #7314 ), #13065, .T. ) ;
#5340=CARTESIAN_POINT ( 'NONE',  ( -167.4745151998187680, 32.15905408292206147, -2.500000000000000000 ) ) ;
#5354=CARTESIAN_POINT ( 'NONE',  ( -73.14061779976039190, 46.33634706135890013, 2.761024190134958811 ) ) ;
#5365=VECTOR ( 'NONE', #3530, 1000.000000000000000 ) ;
#5374=EDGE_CURVE ( 'NONE', #6411, #16333, #15117, .T. ) ;
#5385=VECTOR ( 'NONE', #16974, 1000.000000000000000 ) ;
#5387=LINE ( 'NONE', #11145, #5385 ) ;
#5397=SHAPE_REPRESENTATION ( 'Upper Squeezer Handle Arm', ( #18772 ), #18155 ) ;
#5400=CARTESIAN_POINT ( 'NONE',  ( -81.37351714223066779, 3.066920708278495944, -2.499999999999999112 ) ) ;
#5409=ORIENTED_EDGE ( 'NONE', *, *, #14957, .F. ) ;
#5412=VERTEX_POINT ( 'NONE', #5055 ) ;
#5417=LINE ( 'NONE', #11178, #7654 ) ;
#5439=CARTESIAN_POINT ( 'NONE',  ( 73.09088021254186174, 1.387778780781445676E-14, 110.7545852194966045 ) ) ;
#5451=AXIS2_PLACEMENT_3D ( 'NONE', #15474, #16819, #3702 ) ;
#5487=DIRECTION ( 'NONE',  ( 2.671473304378624222E-16, 0.000000000000000000, 1.000000000000000000 ) ) ;
#5492=CYLINDRICAL_SURFACE ( 'NONE', #11779, 145.0000000000000000 ) ;
#5509=FACE_BOUND ( 'NONE', #3543, .T. ) ;
#5524=ORIENTED_EDGE ( 'NONE', *, *, #16557, .F. ) ;
#5534=ORIENTED_EDGE ( 'NONE', *, *, #5374, .F. ) ;
#5550=DIRECTION ( 'NONE',  ( -1.000000000000000000, 0.000000000000000000, 0.000000000000000000 ) ) ;
#5561=DIRECTION ( 'NONE',  ( -0.000000000000000000, -0.000000000000000000, -1.000000000000000000 ) ) ;
#5595=EDGE_CURVE ( 'NONE', #10837, #3705, #575, .T. ) ;
#5604=ORIENTED_EDGE ( 'NONE', *, *, #13083, .F. ) ;
#5632=B_SPLINE_CURVE_WITH_KNOTS ( 'NONE', 3,
 ( #2305, #16841, #6696, #14157, #3900, #5354, #2408, #12244, #18290, #2508, #9805, #12338, #14057, #16933, #8297, #11011, #5165, #2595, #15573, #1103 ),
 .UNSPECIFIED., .F., .F.,
 ( 4, 2, 2, 2, 2, 2, 2, 2, 2, 4 ),
 ( 4.336808689942017736E-19, 0.0009785997360078372773, 0.001467899604011736617, 0.001957199472015635957, 0.002935799208023399508, 0.003914398944031161759, 0.004892998680038927045, 0.005871598416046690597, 0.006850198152054454148, 0.007828797888062217700 ),
 .UNSPECIFIED. ) ;
#5651=CIRCLE ( 'NONE', #10170, 150.0000000000000284 ) ;
#5660=EDGE_LOOP ( 'NONE', ( #14979, #3913, #3517, #4634 ) ) ;
#5667=CARTESIAN_POINT ( 'NONE',  ( -79.48148684286209686, 1.792690752935663046, 3.092063782402497907 ) ) ;
#5692=EDGE_CURVE ( 'NONE', #17705, #12460, #5101, .T. ) ;
#5695=ADVANCED_FACE ( 'NONE', ( #3332 ), #9136, .T. ) ;
#5704=CARTESIAN_POINT ( 'NONE',  ( -79.05438463828195950, 1.499069270643396345, -3.389939594122236333 ) ) ;
#5726=STYLED_ITEM ( 'NONE', ( #16963 ), #10448 ) ;
#5739=CARTESIAN_POINT ( 'NONE',  ( -172.4977872642596424, 56.55098501587584536, 2.500000000000000000 ) ) ;
#5741=DIRECTION ( 'NONE',  ( -0.000000000000000000, -0.000000000000000000, -1.000000000000000000 ) ) ;
#5751=ORIENTED_EDGE ( 'NONE', *, *, #7442, .T. ) ;
#5754=CARTESIAN_POINT ( 'NONE',  ( -176.1167811578620501, -139.6880237571007513, -2.500000000000000000 ) ) ;
#5758=ORIENTED_EDGE ( 'NONE', *, *, #7293, .T. ) ;
#5773=ORIENTED_EDGE ( 'NONE', *, *, #5318, .T. ) ;
#5791=CARTESIAN_POINT ( 'NONE',  ( -69.99999999999998579, -45.00000000000000711, 25.00000000000000000 ) ) ;
#5822=DIRECTION ( 'NONE',  ( 0.000000000000000000, -0.000000000000000000, -1.000000000000000000 ) ) ;
#5840=CARTESIAN_POINT ( 'NONE',  ( -70.94787397664823914, 45.40332465903016868, -4.449065472295569812 ) ) ;
#5868=AXIS2_PLACEMENT_3D ( 'NONE', #836, #15514, #13890 ) ;
#5878=DIRECTION ( 'NONE',  ( 1.000000000000000000, 0.000000000000000000, 0.000000000000000000 ) ) ;
#5880=EDGE_CURVE ( 'NONE', #15891, #2138, #1181, .T. ) ;
#5889=VERTEX_POINT ( 'NONE', #10671 ) ;
#5903=ORIENTED_EDGE ( 'NONE', *, *, #10465, .F. ) ;
#5908=DIRECTION ( 'NONE',  ( -0.000000000000000000, -0.000000000000000000, 1.000000000000000000 ) ) ;
#5916=CARTESIAN_POINT ( 'NONE',  ( -174.6158025762232171, 55.77168144464769028, -4.051035741711864091 ) ) ;
#5917=CARTESIAN_POINT ( 'NONE',  ( -69.99999999999998579, -45.00000000000000711, 20.00000000000001776 ) ) ;
#5918=EDGE_CURVE ( 'NONE', #7914, #753, #830, .T. ) ;
#5926=APPLICATION_CONTEXT ( 'automotive_design' ) ;
#5957=CARTESIAN_POINT ( 'NONE',  ( -76.90911978745816668, 1.387778780781445676E-14, -7.500000000000000000 ) ) ;
#5967=VECTOR ( 'NONE', #9185, 1000.000000000000000 ) ;
#5995=ORIENTED_EDGE ( 'NONE', *, *, #7303, .F. ) ;
#6003=CARTESIAN_POINT ( 'NONE',  ( -174.4298649410498854, 55.90939826654244627, 3.724467847532853426 ) ) ;
#6004=CARTESIAN_POINT ( 'NONE',  ( -62.00000000000000000, 0.000000000000000000, -25.00000000000000000 ) ) ;
#6007=CARTESIAN_POINT ( 'NONE',  ( -71.80233157044055758, 45.76690022515197853, -3.524781480481925744 ) ) ;
#6028=EDGE_CURVE ( 'NONE', #15891, #3230, #13185, .T. ) ;
#6031=DIRECTION ( 'NONE',  ( -1.000000000000000000, 0.000000000000000000, 0.000000000000000000 ) ) ;
#6038=AXIS2_PLACEMENT_3D ( 'NONE', #15291, #8090, #12620 ) ;
#6057=FACE_OUTER_BOUND ( 'NONE', #15034, .T. ) ;
#6059=CARTESIAN_POINT ( 'NONE',  ( 73.09088021254186174, 1.387778780781445676E-14, 2.500000000000000444 ) ) ;
#6073=ORIENTED_EDGE ( 'NONE', *, *, #2903, .T. ) ;
#6087=AXIS2_PLACEMENT_3D ( 'NONE', #7909, #4944, #17898 ) ;
#6088=EDGE_CURVE ( 'NONE', #15023, #7569, #15610, .T. ) ;
#6090=ORIENTED_EDGE ( 'NONE', *, *, #5044, .T. ) ;
#6098=EDGE_LOOP ( 'NONE', ( #17603, #8589, #14047 ) ) ;
#6099=CARTESIAN_POINT ( 'NONE',  ( -173.0810787726268245, 56.45151975169574143, -2.500000000000000000 ) ) ;
#6114=CARTESIAN_POINT ( 'NONE',  ( -79.20163718375225415, 48.91533818955501545, -2.500000000000000000 ) ) ;
#6129=PLANE ( 'NONE',  #8516 ) ;
#6150=DIRECTION ( 'NONE',  ( 1.000000000000000000, 0.000000000000000000, 0.000000000000000000 ) ) ;
#6158=EDGE_LOOP ( 'NONE', ( #1258, #6201, #7744 ) ) ;
#6165=LINE ( 'NONE', #9183, #5117 ) ;
#6168=ORIENTED_EDGE ( 'NONE', *, *, #15060, .T. ) ;
#6197=ADVANCED_FACE ( 'NONE', ( #15868 ), #14447, .F. ) ;
#6201=ORIENTED_EDGE ( 'NONE', *, *, #7223, .T. ) ;
#6211=DIRECTION ( 'NONE',  ( -0.9857117110570272622, -0.1684411549622826243, 2.137303368083796319E-18 ) ) ;
#6236=CARTESIAN_POINT ( 'NONE',  ( -69.99999999999998579, -45.00000000000000711, -19.99999999999999645 ) ) ;
#6238=AXIS2_PLACEMENT_3D ( 'NONE', #7167, #5741, #10163 ) ;
#6251=FACE_OUTER_BOUND ( 'NONE', #16611, .T. ) ;
#6260=CARTESIAN_POINT ( 'NONE',  ( -172.7326993491721225, 43.83249341393818810, 9.951701414186830458E-16 ) ) ;
#6271=EDGE_CURVE ( 'NONE', #15200, #753, #10427, .T. ) ;
#6288=EDGE_LOOP ( 'NONE', ( #15699, #15812, #6461, #4492 ) ) ;
#6296=EDGE_CURVE ( 'NONE', #13205, #4027, #17669, .T. ) ;
#6306=ORIENTED_EDGE ( 'NONE', *, *, #7990, .F. ) ;
#6308=CARTESIAN_POINT ( 'NONE',  ( -175.0988807681447383, 56.35851375132025254, 2.556294622946508611E-15 ) ) ;
#6338=DIRECTION ( 'NONE',  ( 3.816390434826605238E-17, 0.000000000000000000, -1.000000000000000000 ) ) ;
#6365=DIRECTION ( 'NONE',  ( -0.000000000000000000, -0.000000000000000000, -1.000000000000000000 ) ) ;
#6377=AXIS2_PLACEMENT_3D ( 'NONE', #12131, #9217, #7800 ) ;
#6403=CARTESIAN_POINT ( 'NONE',  ( -73.42100199588526266, 46.45565180342956779, -2.660647884740717561 ) ) ;
#6411=VERTEX_POINT ( 'NONE', #1916 ) ;
#6413=DIRECTION ( 'NONE',  ( 1.000000000000000000, 0.000000000000000000, 0.000000000000000000 ) ) ;
#6416=AXIS2_PLACEMENT_3D ( 'NONE', #18472, #17398, #2859 ) ;
#6430=EDGE_LOOP ( 'NONE', ( #12252, #18428 ) ) ;
#6434=CARTESIAN_POINT ( 'NONE',  ( -62.00000000000000000, 0.000000000000000000, -20.00000000000000000 ) ) ;
#6437=ORIENTED_EDGE ( 'NONE', *, *, #13859, .T. ) ;
#6452=DIRECTION ( 'NONE',  ( 0.000000000000000000, 0.000000000000000000, 1.000000000000000000 ) ) ;
#6461=ORIENTED_EDGE ( 'NONE', *, *, #359, .F. ) ;
#6463=PLANE ( 'NONE',  #13657 ) ;
#6466=DIRECTION ( 'NONE',  ( -0.9826218788918642533, -0.1856185419698762884, 0.000000000000000000 ) ) ;
#6475=ORIENTED_EDGE ( 'NONE', *, *, #3561, .T. ) ;
#6488=EDGE_CURVE ( 'NONE', #13205, #2144, #8365, .T. ) ;
#6498=CARTESIAN_POINT ( 'NONE',  ( -174.3141932433752004, 55.97754034394239397, -3.563338245596195719 ) ) ;
#6501=DIRECTION ( 'NONE',  ( -0.000000000000000000, -0.000000000000000000, -1.000000000000000000 ) ) ;
#6514=ORIENTED_EDGE ( 'NONE', *, *, #4514, .F. ) ;
#6518=ORIENTED_EDGE ( 'NONE', *, *, #4723, .T. ) ;
#6523=DIRECTION ( 'NONE',  ( 1.000000000000000000, 0.000000000000000000, 0.000000000000000000 ) ) ;
#6536=CARTESIAN_POINT ( 'NONE',  ( -70.00000000000000000, 44.99999999999999289, 25.00000000000000000 ) ) ;
#6551=ORIENTED_EDGE ( 'NONE', *, *, #17754, .F. ) ;
#6557=ADVANCED_FACE ( 'NONE', ( #2481, #16713, #2276 ), #3690, .T. ) ;
#6567=SURFACE_STYLE_USAGE ( .BOTH. , #13734 ) ;
#6571=AXIS2_PLACEMENT_3D ( 'NONE', #7564, #361, #10301 ) ;
#6574=ORIENTED_EDGE ( 'NONE', *, *, #17615, .T. ) ;
#6578=CARTESIAN_POINT ( 'NONE',  ( -169.7775681651189359, 31.94775928504250828, -3.566331213966874802 ) ) ;
#6589=ORIENTED_EDGE ( 'NONE', *, *, #6732, .F. ) ;
#6620=LINE ( 'NONE', #13700, #18712 ) ;
#6623=VERTEX_POINT ( 'NONE', #3593 ) ;
#6629=CARTESIAN_POINT ( 'NONE',  ( -137.7298645655810390, -88.63485219053825404, -2.500000000000000000 ) ) ;
#6638=EDGE_CURVE ( 'NONE', #14394, #18427, #16605, .T. ) ;
#6647=ORIENTED_EDGE ( 'NONE', *, *, #7816, .T. ) ;
#6651=DIRECTION ( 'NONE',  ( 0.1856185419698760941, -0.9826218788918640312, 0.000000000000000000 ) ) ;
#6660=ORIENTED_EDGE ( 'NONE', *, *, #14355, .F. ) ;
#6676=DIRECTION ( 'NONE',  ( -0.3915338189555022108, -0.9201637183752248150, 0.000000000000000000 ) ) ;
#6696=CARTESIAN_POINT ( 'NONE',  ( -74.01821019817211322, 46.70976659135642706, 2.532235937273572546 ) ) ;
#6700=VECTOR ( 'NONE', #8705, 1000.000000000000000 ) ;
#6732=EDGE_CURVE ( 'NONE', #15023, #17089, #2731, .T. ) ;
#6740=VECTOR ( 'NONE', #9545, 1000.000000000000227 ) ;
#6749=CARTESIAN_POINT ( 'NONE',  ( -70.00000000000000000, 44.99999999999999289, 110.7545852194966045 ) ) ;
#6768=DIRECTION ( 'NONE',  ( 0.000000000000000000, 0.000000000000000000, 1.000000000000000000 ) ) ;
#6772=DIRECTION ( 'NONE',  ( -0.9539392014169452150, 0.3000000000000013212, -0.000000000000000000 ) ) ;
#6775=VERTEX_POINT ( 'NONE', #5704 ) ;
#6789=AXIS2_PLACEMENT_3D ( 'NONE', #1128, #4024, #11317 ) ;
#6797=CARTESIAN_POINT ( 'NONE',  ( 5.481473465377021625, 12.88229205725314763, -25.00000000000000000 ) ) ;
#6804=ORIENTED_EDGE ( 'NONE', *, *, #2884, .F. ) ;
#6822=EDGE_LOOP ( 'NONE', ( #11394, #15808, #4959, #12412, #9912, #4907, #14046, #6551, #3842, #17985 ) ) ;
#6823=DIRECTION ( 'NONE',  ( -0.000000000000000000, -0.000000000000000000, -1.000000000000000000 ) ) ;
#6826=EDGE_LOOP ( 'NONE', ( #3695, #17374, #13877, #10071 ) ) ;
#6829=DIRECTION ( 'NONE',  ( -0.000000000000000000, -0.000000000000000000, -1.000000000000000000 ) ) ;
#6849=EDGE_CURVE ( 'NONE', #4027, #10083, #5028, .T. ) ;
#6897=ORIENTED_EDGE ( 'NONE', *, *, #10465, .T. ) ;
#6922=DIRECTION ( 'NONE',  ( -0.000000000000000000, -0.000000000000000000, -1.000000000000000000 ) ) ;
#6931=ORIENTED_EDGE ( 'NONE', *, *, #9658, .T. ) ;
#6934=TOROIDAL_SURFACE ( 'NONE', #9324, 12.83663829214476770, 3.000000000000000000 ) ;
#6940=FACE_OUTER_BOUND ( 'NONE', #17475, .T. ) ;
#6943=CARTESIAN_POINT ( 'NONE',  ( -81.87192997736541145, 3.395211045985502274, 2.500000000000000000 ) ) ;
#6960=ORIENTED_EDGE ( 'NONE', *, *, #9156, .T. ) ;
#6961=DIRECTION ( 'NONE',  ( -0.3000000000000046518, 0.9539392014169442158, 0.000000000000000000 ) ) ;
#6975=EDGE_LOOP ( 'NONE', ( #16868, #17786, #13752 ) ) ;
#6981=UNCERTAINTY_MEASURE_WITH_UNIT (LENGTH_MEASURE( 1.000000000000000082E-05 ), #18508, 'distance_accuracy_value', 'NONE');
#6983=DIRECTION ( 'NONE',  ( 0.1856185419698755945, -0.9826218788918641422, 0.000000000000000000 ) ) ;
#6986=AXIS2_PLACEMENT_3D ( 'NONE', #14877, #11908, #17753 ) ;
#6988=DIRECTION ( 'NONE',  ( 3.816390434826605238E-17, 0.000000000000000000, -1.000000000000000000 ) ) ;
#6993=AXIS2_PLACEMENT_3D ( 'NONE', #998, #3879, #9706 ) ;
#7000=CARTESIAN_POINT ( 'NONE',  ( 5.481473465377026955, -12.88229205725314763, 25.00000000000000000 ) ) ;
#7001=EDGE_LOOP ( 'NONE', ( #5092, #10155, #5120 ) ) ;
#7017=CARTESIAN_POINT ( 'NONE',  ( -71.90911978745813826, 1.387778780781445676E-14, -19.99999999999999645 ) ) ;
#7018=CARTESIAN_POINT ( 'NONE',  ( -62.00000000000000000, 0.000000000000000000, -20.00000000000000000 ) ) ;
#7043=DIRECTION ( 'NONE',  ( -0.9826218788918641422, -0.1856185419698762606, 0.000000000000000000 ) ) ;
#7047=DIRECTION ( 'NONE',  ( -0.000000000000000000, -0.000000000000000000, -1.000000000000000000 ) ) ;
#7050=ORIENTED_EDGE ( 'NONE', *, *, #16699, .F. ) ;
#7053=VECTOR ( 'NONE', #6829, 1000.000000000000000 ) ;
#7071=ORIENTED_EDGE ( 'NONE', *, *, #18192, .F. ) ;
#7075=LINE ( 'NONE', #9881, #10929 ) ;
#7105=EDGE_LOOP ( 'NONE', ( #2415, #1410, #10152, #326, #12219 ) ) ;
#7120=CARTESIAN_POINT ( 'NONE',  ( 73.09088021254186174, 1.387778780781445676E-14, 25.00000000000000000 ) ) ;
#7165=CARTESIAN_POINT ( 'NONE',  ( -173.9176162982875269, 56.15916356109917729, 3.150553392547033482 ) ) ;
#7167=CARTESIAN_POINT ( 'NONE',  ( 0.000000000000000000, 0.000000000000000000, 25.00000000000000000 ) ) ;
#7186=VERTEX_POINT ( 'NONE', #7444 ) ;
#7210=AXIS2_PLACEMENT_3D ( 'NONE', #10363, #3429, #4768 ) ;
#7223=EDGE_CURVE ( 'NONE', #15023, #2144, #4216, .T. ) ;
#7232=CARTESIAN_POINT ( 'NONE',  ( -77.11857033228203306, -1.071618245585014506, -6.007947165629304642 ) ) ;
#7239=AXIS2_PLACEMENT_3D ( 'NONE', #3959, #9934, #14315 ) ;
#7254=CIRCLE ( 'NONE', #12661, 2.200000000000000178 ) ;
#7257=DIRECTION ( 'NONE',  ( -0.000000000000000000, -0.000000000000000000, -1.000000000000000000 ) ) ;
#7263=CARTESIAN_POINT ( 'NONE',  ( -70.61186533023291645, 45.26035146208064219, -4.992628012786330949 ) ) ;
#7273=AXIS2_PLACEMENT_3D ( 'NONE', #1280, #5822, #13092 ) ;
#7279=CARTESIAN_POINT ( 'NONE',  ( 0.000000000000000000, 0.000000000000000000, -25.00000000000000000 ) ) ;
#7288=EDGE_CURVE ( 'NONE', #13047, #15200, #4864, .T. ) ;
#7289=CARTESIAN_POINT ( 'NONE',  ( -81.37336115545215875, 3.066817964230565963, 2.499999999999999556 ) ) ;
#7293=EDGE_CURVE ( 'NONE', #14073, #56, #15468, .T. ) ;
#7298=ORIENTED_EDGE ( 'NONE', *, *, #8750, .T. ) ;
#7303=EDGE_CURVE ( 'NONE', #8040, #11020, #16687, .T. ) ;
#7314=FACE_OUTER_BOUND ( 'NONE', #14316, .T. ) ;
#7318=ORIENTED_EDGE ( 'NONE', *, *, #17546, .T. ) ;
#7329=ADVANCED_FACE ( 'NONE', ( #1846 ), #12152, .F. ) ;
#7336=ORIENTED_EDGE ( 'NONE', *, *, #4626, .F. ) ;
#7359=FACE_OUTER_BOUND ( 'NONE', #142, .T. ) ;
#7402=EDGE_LOOP ( 'NONE', ( #13818, #11359 ) ) ;
#7404=ORIENTED_EDGE ( 'NONE', *, *, #12484, .T. ) ;
#7422=ADVANCED_FACE ( 'NONE', ( #1194 ), #14052, .F. ) ;
#7435=DIRECTION ( 'NONE',  ( 1.000000000000000000, 0.000000000000000000, 0.000000000000000000 ) ) ;
#7442=EDGE_CURVE ( 'NONE', #4836, #15547, #11005, .T. ) ;
#7444=CARTESIAN_POINT ( 'NONE',  ( -65.23030399291525327, 43.49999999999997868, 20.00000000000001776 ) ) ;
#7449=DIRECTION ( 'NONE',  ( -0.9201637183752249260, -0.3915338189555018777, -3.511704013281690003E-17 ) ) ;
#7455=CARTESIAN_POINT ( 'NONE',  ( -172.7326993491721225, 43.83249341393818810, 9.951701414186830458E-16 ) ) ;
#7456=DIRECTION ( 'NONE',  ( 0.000000000000000000, 0.000000000000000000, 1.000000000000000000 ) ) ;
#7473=DIRECTION ( 'NONE',  ( 0.000000000000000000, 0.000000000000000000, 1.000000000000000000 ) ) ;
#7497=ORIENTED_EDGE ( 'NONE', *, *, #14085, .F. ) ;
#7516=CIRCLE ( 'NONE', #16296, 2.200000000000000622 ) ;
#7520=EDGE_CURVE ( 'NONE', #10837, #4610, #7075, .T. ) ;
#7538=AXIS2_PLACEMENT_3D ( 'NONE', #14907, #12134, #4936 ) ;
#7540=DIRECTION ( 'NONE',  ( -0.9539392014169452150, 0.3000000000000013212, 2.548423110585632720E-16 ) ) ;
#7544=VECTOR ( 'NONE', #14224, 1000.000000000000227 ) ;
#7545=ADVANCED_FACE ( 'NONE', ( #130 ), #18747, .F. ) ;
#7564=CARTESIAN_POINT ( 'NONE',  ( 73.09088021254186174, 1.387778780781445676E-14, -25.00000000000000000 ) ) ;
#7569=VERTEX_POINT ( 'NONE', #14626 ) ;
#7576=AXIS2_PLACEMENT_3D ( 'NONE', #18418, #5487, #9757 ) ;
#7583=ADVANCED_FACE ( 'NONE', ( #11383 ), #16046, .F. ) ;
#7602=ORIENTED_EDGE ( 'NONE', *, *, #12410, .T. ) ;
#7604=VECTOR ( 'NONE', #3930, 1000.000000000000000 ) ;
#7621=EDGE_LOOP ( 'NONE', ( #3492, #8695, #4045, #4111, #13664 ) ) ;
#7622=CARTESIAN_POINT ( 'NONE',  ( -70.00000000000001421, 44.99999999999998579, -7.500000000000000000 ) ) ;
#7626=DIRECTION ( 'NONE',  ( 1.000000000000000000, 0.000000000000000000, 0.000000000000000000 ) ) ;
#7654=VECTOR ( 'NONE', #9780, 1000.000000000000227 ) ;
#7669=DIRECTION ( 'NONE',  ( 3.816390434826605238E-17, 0.000000000000000000, -1.000000000000000000 ) ) ;
#7671=CARTESIAN_POINT ( 'NONE',  ( -65.37641414873196766, 43.03264333350144710, 20.00000000000001066 ) ) ;
#7699=ORIENTED_EDGE ( 'NONE', *, *, #11873, .F. ) ;
#7703=ORIENTED_EDGE ( 'NONE', *, *, #3123, .T. ) ;
#7729=EDGE_CURVE ( 'NONE', #8619, #3230, #13523, .T. ) ;
#7744=ORIENTED_EDGE ( 'NONE', *, *, #10473, .F. ) ;
#7752=CARTESIAN_POINT ( 'NONE',  ( -70.00000000000000000, 44.99999999999999289, 110.7545852194966045 ) ) ;
#7784=CIRCLE ( 'NONE', #6571, 150.0000000000000284 ) ;
#7800=DIRECTION ( 'NONE',  ( 1.000000000000000000, 0.000000000000000000, -0.000000000000000000 ) ) ;
#7802=CARTESIAN_POINT ( 'NONE',  ( -172.7326993491721225, 43.83249341393818810, 9.951701414186830458E-16 ) ) ;
#7816=EDGE_CURVE ( 'NONE', #56, #15303, #7864, .T. ) ;
#7822=CARTESIAN_POINT ( 'NONE',  ( -59.79999999999999716, 0.000000000000000000, 20.00000000000001776 ) ) ;
#7834=AXIS2_PLACEMENT_3D ( 'NONE', #7802, #10716, #10446 ) ;
#7835=ORIENTED_EDGE ( 'NONE', *, *, #3581, .F. ) ;
#7841=DIRECTION ( 'NONE',  ( 0.9826218788918644753, 0.1856185419698747896, 0.000000000000000000 ) ) ;
#7863=AXIS2_PLACEMENT_3D ( 'NONE', #8950, #15975, #15881 ) ;
#7864=LINE ( 'NONE', #18430, #7053 ) ;
#7867=CARTESIAN_POINT ( 'NONE',  ( -69.99999999999998579, -45.00000000000000711, 25.00000000000000000 ) ) ;
#7890=ADVANCED_FACE ( 'NONE', ( #18126 ), #671, .F. ) ;
#7899=CARTESIAN_POINT ( 'NONE',  ( -70.00000000000000000, 44.99999999999999289, 25.00000000000000000 ) ) ;
#7900=CARTESIAN_POINT ( 'NONE',  ( 5.481473465377015408, 12.88229205725314408, 20.00000000000000000 ) ) ;
#7909=CARTESIAN_POINT ( 'NONE',  ( 0.000000000000000000, 0.000000000000000000, 25.00000000000000000 ) ) ;
#7912=CARTESIAN_POINT ( 'NONE',  ( -169.9035932455946636, 31.96784544054909816, 3.719291248522914373 ) ) ;
#7913=CARTESIAN_POINT ( 'NONE',  ( -173.9130733970031883, 56.16092972190472210, -3.146712427857100813 ) ) ;
#7914=VERTEX_POINT ( 'NONE', #18236 ) ;
#7943=( NAMED_UNIT ( * ) SI_UNIT ( $, .STERADIAN. ) SOLID_ANGLE_UNIT ( ) );
#7953=ORIENTED_EDGE ( 'NONE', *, *, #1331, .F. ) ;
#7954=VERTEX_POINT ( 'NONE', #12571 ) ;
#7959=PLANE ( 'NONE',  #7239 ) ;
#7964=DIRECTION ( 'NONE',  ( -0.000000000000000000, -0.000000000000000000, -1.000000000000000000 ) ) ;
#7978=SURFACE_STYLE_FILL_AREA ( #2196 ) ;
#7990=EDGE_CURVE ( 'NONE', #9050, #12460, #12341, .T. ) ;
#7997=CARTESIAN_POINT ( 'NONE',  ( -172.0951522251743029, 56.61964399677355431, -2.500000000000000000 ) ) ;
#8022=FILL_AREA_STYLE_COLOUR ( '', #3861 ) ;
#8032=ORIENTED_EDGE ( 'NONE', *, *, #9658, .F. ) ;
#8040=VERTEX_POINT ( 'NONE', #13051 ) ;
#8047=CARTESIAN_POINT ( 'NONE',  ( 0.000000000000000000, 0.000000000000000000, 25.00000000000000000 ) ) ;
#8067=CARTESIAN_POINT ( 'NONE',  ( -69.99999999999998579, -45.00000000000000711, 110.7545852194966045 ) ) ;
#8070=CARTESIAN_POINT ( 'NONE',  ( 5.481473465377026955, -12.88229205725314763, -25.00000000000000000 ) ) ;
#8071=CARTESIAN_POINT ( 'NONE',  ( -70.00000000000000000, 44.99999999999999289, -19.99999999999999645 ) ) ;
#8078=ORIENTED_EDGE ( 'NONE', *, *, #10037, .F. ) ;
#8084=CIRCLE ( 'NONE', #10783, 2.200000000000000622 ) ;
#8090=DIRECTION ( 'NONE',  ( 0.000000000000000000, 0.000000000000000000, 1.000000000000000000 ) ) ;
#8124=CARTESIAN_POINT ( 'NONE',  ( -174.8673125818257006, 55.13264502119463373, 5.500000000000001776 ) ) ;
#8137=ORIENTED_EDGE ( 'NONE', *, *, #7303, .T. ) ;
#8151=DIRECTION ( 'NONE',  ( 0.1856185419698760941, -0.9826218788918640312, 0.000000000000000000 ) ) ;
#8157=FACE_OUTER_BOUND ( 'NONE', #14229, .T. ) ;
#8177=CARTESIAN_POINT ( 'NONE',  ( 5.481473465377026955, -12.88229205725314763, 25.00000000000000000 ) ) ;
#8216=EDGE_CURVE ( 'NONE', #5889, #897, #14576, .T. ) ;
#8219=ORIENTED_EDGE ( 'NONE', *, *, #16094, .T. ) ;
#8241=DIRECTION ( 'NONE',  ( -2.671473304378624222E-16, -0.000000000000000000, -1.000000000000000000 ) ) ;
#8260=CARTESIAN_POINT ( 'NONE',  ( -70.00000000000000000, 44.99999999999999289, -19.99999999999998934 ) ) ;
#8267=ORIENTED_EDGE ( 'NONE', *, *, #15968, .T. ) ;
#8279=PLANE ( 'NONE',  #2121 ) ;
#8284=CARTESIAN_POINT ( 'NONE',  ( -62.00000000000000000, 0.000000000000000000, 20.00000000000001776 ) ) ;
#8292=EDGE_CURVE ( 'NONE', #18427, #4539, #7784, .T. ) ;
#8295=EDGE_CURVE ( 'NONE', #11597, #11722, #2927, .T. ) ;
#8297=CARTESIAN_POINT ( 'NONE',  ( -70.47070042840788062, 45.20028515864974850, 5.277796196381517646 ) ) ;
#8309=DIRECTION ( 'NONE',  ( -0.000000000000000000, -0.000000000000000000, -1.000000000000000000 ) ) ;
#8335=ORIENTED_EDGE ( 'NONE', *, *, #16291, .T. ) ;
#8340=DIRECTION ( 'NONE',  ( 0.1856185419698755945, -0.9826218788918641422, 0.000000000000000000 ) ) ;
#8365=B_SPLINE_CURVE_WITH_KNOTS ( 'NONE', 3,
 ( #4567, #6099, #496, #11843 ),
 .UNSPECIFIED., .F., .F.,
 ( 4, 4 ),
 ( 0.000000000000000000, 0.003000475340473865958 ),
 .UNSPECIFIED. ) ;
#8413=CARTESIAN_POINT ( 'NONE',  ( -77.11859967870812227, -1.071530569176025516, 6.007857748507488438 ) ) ;
#8420=CIRCLE ( 'NONE', #2664, 15.83618137761394173 ) ;
#8454=CARTESIAN_POINT ( 'NONE',  ( -176.1167811578620501, -139.6880237571007513, -2.500000000000000000 ) ) ;
#8481=CIRCLE ( 'NONE', #12680, 2.200000000000000178 ) ;
#8486=CIRCLE ( 'NONE', #1238, 2.200000000000000622 ) ;
#8516=AXIS2_PLACEMENT_3D ( 'NONE', #17708, #4678, #3249 ) ;
#8538=VECTOR ( 'NONE', #11530, 1000.000000000000000 ) ;
#8540=CARTESIAN_POINT ( 'NONE',  ( -70.00000000000000000, 44.99999999999999289, -25.00000000000000000 ) ) ;
#8548=ORIENTED_EDGE ( 'NONE', *, *, #17546, .F. ) ;
#8556=CARTESIAN_POINT ( 'NONE',  ( -77.24748271550588186, -0.7169195224846902637, -5.646145272226924305 ) ) ;
#8559=CARTESIAN_POINT ( 'NONE',  ( -2.200000000000000178, 0.000000000000000000, 25.00000000000000000 ) ) ;
#8572=ORIENTED_EDGE ( 'NONE', *, *, #6488, .T. ) ;
#8575=VERTEX_POINT ( 'NONE', #18599 ) ;
#8589=ORIENTED_EDGE ( 'NONE', *, *, #4950, .T. ) ;
#8603=DIRECTION ( 'NONE',  ( 0.9201637183752250371, -0.3915338189555017667, 3.511704013281690619E-17 ) ) ;
#8619=VERTEX_POINT ( 'NONE', #4845 ) ;
#8626=DIRECTION ( 'NONE',  ( 2.671473304378624222E-16, 0.000000000000000000, 1.000000000000000000 ) ) ;
#8642=LINE ( 'NONE', #17295, #13596 ) ;
#8650=CYLINDRICAL_SURFACE ( 'NONE', #11768, 3.000000000000003109 ) ;
#8659=DIRECTION ( 'NONE',  ( -0.000000000000000000, -0.000000000000000000, 1.000000000000000000 ) ) ;
#8663=VECTOR ( 'NONE', #13062, 1000.000000000000114 ) ;
#8667=CARTESIAN_POINT ( 'NONE',  ( -172.0951522251743029, 56.61964399677356141, 2.500000000000000000 ) ) ;
#8669=CARTESIAN_POINT ( 'NONE',  ( -70.15512743057031742, 45.06600742248694047, -6.205119912480675737 ) ) ;
#8693=CIRCLE ( 'NONE', #15344, 2.200000000000007283 ) ;
#8695=ORIENTED_EDGE ( 'NONE', *, *, #14697, .F. ) ;
#8700=CARTESIAN_POINT ( 'NONE',  ( -167.4745151998187680, 32.15905408292213252, 2.500000000000000000 ) ) ;
#8705=DIRECTION ( 'NONE',  ( 0.000000000000000000, 0.000000000000000000, 1.000000000000000000 ) ) ;
#8724=EDGE_LOOP ( 'NONE', ( #4788, #10507 ) ) ;
#8728=CARTESIAN_POINT ( 'NONE',  ( -78.35787276487999975, 0.9448187065377893212, -3.952829652586226761 ) ) ;
#8739=VECTOR ( 'NONE', #18335, 1000.000000000000000 ) ;
#8746=ORIENTED_EDGE ( 'NONE', *, *, #17782, .T. ) ;
#8750=EDGE_CURVE ( 'NONE', #14167, #12815, #5417, .T. ) ;
#8766=ORIENTED_EDGE ( 'NONE', *, *, #3787, .T. ) ;
#8769=MANIFOLD_SOLID_BREP ( 'Move Face1', #18776 ) ;
#8782=EDGE_LOOP ( 'NONE', ( #6073, #6437, #5751, #18488, #17258 ) ) ;
#8783=ORIENTED_EDGE ( 'NONE', *, *, #17715, .T. ) ;
#8791=ORIENTED_EDGE ( 'NONE', *, *, #15456, .F. ) ;
#8826=DIRECTION ( 'NONE',  ( 1.000000000000000000, 5.329070518200749027E-15, -2.631994239413086031E-16 ) ) ;
#8835=CARTESIAN_POINT ( 'NONE',  ( -65.37641414873195345, -43.03264333350145421, 20.00000000000001421 ) ) ;
#8849=CONICAL_SURFACE ( 'NONE', #17954, 12.74754878398197633, 0.01745329251994333364 ) ;
#8859=CARTESIAN_POINT ( 'NONE',  ( -71.56969528596198415, 45.66791243518527921, -3.731434853903564886 ) ) ;
#8864=ADVANCED_FACE ( 'NONE', ( #4167 ), #14606, .F. ) ;
#8866=COLOUR_RGB ( '', 0.08235294, 0.09019608, 0.10196078) ;
#8870=EDGE_CURVE ( 'NONE', #6775, #15850, #10541, .T. ) ;
#8877=CARTESIAN_POINT ( 'NONE',  ( 0.000000000000000000, 0.000000000000000000, 25.00000000000000000 ) ) ;
#8882=DIRECTION ( 'NONE',  ( 1.000000000000000000, 0.000000000000000000, 0.000000000000000000 ) ) ;
#8950=CARTESIAN_POINT ( 'NONE',  ( -172.7326993491721225, 43.83249341393818810, 9.951701414186830458E-16 ) ) ;
#8979=EDGE_CURVE ( 'NONE', #113, #4333, #13525, .T. ) ;
#8984=CIRCLE ( 'NONE', #14130, 145.0000000000000284 ) ;
#9006=DIRECTION ( 'NONE',  ( -0.000000000000000000, -0.000000000000000000, 1.000000000000000000 ) ) ;
#9012=ORIENTED_EDGE ( 'NONE', *, *, #17803, .F. ) ;
#9050=VERTEX_POINT ( 'NONE', #1064 ) ;
#9130=DIRECTION ( 'NONE',  ( -0.3915338189555018222, -0.9201637183752250371, 0.000000000000000000 ) ) ;
#9136=CYLINDRICAL_SURFACE ( 'NONE', #7538, 13.99999999999999822 ) ;
#9137=AXIS2_PLACEMENT_3D ( 'NONE', #13099, #1646, #9977 ) ;
#9141=VERTEX_POINT ( 'NONE', #16983 ) ;
#9156=EDGE_CURVE ( 'NONE', #16919, #11811, #9798, .T. ) ;
#9168=EDGE_LOOP ( 'NONE', ( #8032, #229, #9627, #3991 ) ) ;
#9183=CARTESIAN_POINT ( 'NONE',  ( -70.00000000000001421, -45.00000000000001421, 20.00000000000001776 ) ) ;
#9185=DIRECTION ( 'NONE',  ( -0.000000000000000000, -0.000000000000000000, -1.000000000000000000 ) ) ;
#9206=FACE_OUTER_BOUND ( 'NONE', #4215, .T. ) ;
#9217=DIRECTION ( 'NONE',  ( 0.000000000000000000, 0.000000000000000000, 1.000000000000000000 ) ) ;
#9223=DIRECTION ( 'NONE',  ( 1.000000000000000000, 0.000000000000000000, 0.000000000000000000 ) ) ;
#9244=ADVANCED_FACE ( 'NONE', ( #14484 ), #13054, .T. ) ;
#9255=CARTESIAN_POINT ( 'NONE',  ( 73.09088021254186174, 1.387778780781445676E-14, 25.00000000000000000 ) ) ;
#9256=DIRECTION ( 'NONE',  ( 0.1856185419698760941, -0.9826218788918640312, 0.000000000000000000 ) ) ;
#9261=CARTESIAN_POINT ( 'NONE',  ( -70.00000000000000000, 44.99999999999999289, 7.500000000000007105 ) ) ;
#9264=ORIENTED_EDGE ( 'NONE', *, *, #7442, .F. ) ;
#9266=DIRECTION ( 'NONE',  ( -0.000000000000000000, -0.000000000000000000, -1.000000000000000000 ) ) ;
#9277=FACE_OUTER_BOUND ( 'NONE', #8782, .T. ) ;
#9283=DIRECTION ( 'NONE',  ( -0.000000000000000000, -0.000000000000000000, -1.000000000000000000 ) ) ;
#9314=CARTESIAN_POINT ( 'NONE',  ( -64.20000000000000284, 2.694222958124175527E-16, 20.00000000000001776 ) ) ;
#9324=AXIS2_PLACEMENT_3D ( 'NONE', #10697, #6466, #12199 ) ;
#9327=LINE ( 'NONE', #11870, #13898 ) ;
#9337=ORIENTED_EDGE ( 'NONE', *, *, #1770, .T. ) ;
#9348=ADVANCED_FACE ( 'NONE', ( #14668 ), #3456, .T. ) ;
#9379=DIRECTION ( 'NONE',  ( -0.000000000000000000, -0.000000000000000000, -1.000000000000000000 ) ) ;
#9390=LINE ( 'NONE', #6749, #912 ) ;
#9426=AXIS2_PLACEMENT_3D ( 'NONE', #2073, #3669, #10965 ) ;
#9430=CARTESIAN_POINT ( 'NONE',  ( -70.00000000000002842, 45.00000000000000000, 20.00000000000001776 ) ) ;
#9431=FACE_OUTER_BOUND ( 'NONE', #7105, .T. ) ;
#9445=ADVANCED_FACE ( 'NONE', ( #4700 ), #3413, .T. ) ;
#9469=ADVANCED_FACE ( 'NONE', ( #18312 ), #10750, .F. ) ;
#9477=CARTESIAN_POINT ( 'NONE',  ( 2.200000000000000178, 2.694222958124177006E-16, -19.99999999999999645 ) ) ;
#9490=DIRECTION ( 'NONE',  ( 1.000000000000000000, 0.000000000000000000, -0.000000000000000000 ) ) ;
#9497=( LENGTH_UNIT ( ) NAMED_UNIT ( * ) SI_UNIT ( .MILLI., .METRE. ) );
#9505=ORIENTED_EDGE ( 'NONE', *, *, #8295, .F. ) ;
#9518=CARTESIAN_POINT ( 'NONE',  ( -167.8715234159095928, 32.08088783854852011, 2.520603730400378772 ) ) ;
#9540=ORIENTED_EDGE ( 'NONE', *, *, #4723, .F. ) ;
#9544=ORIENTED_EDGE ( 'NONE', *, *, #3561, .F. ) ;
#9545=DIRECTION ( 'NONE',  ( -0.1856185419698762329, 0.9826218788918640312, -0.000000000000000000 ) ) ;
#9560=AXIS2_PLACEMENT_3D ( 'NONE', #12402, #18248, #8151 ) ;
#9584=ADVANCED_FACE ( 'NONE', ( #13696 ), #426, .F. ) ;
#9587=CIRCLE ( 'NONE', #13824, 145.0000000000000284 ) ;
#9588=CARTESIAN_POINT ( 'NONE',  ( -70.00000000000000000, 44.99999999999999289, 20.00000000000002132 ) ) ;
#9615=FACE_BOUND ( 'NONE', #8724, .T. ) ;
#9617=ADVANCED_FACE ( 'NONE', ( #14082 ), #14182, .F. ) ;
#9627=ORIENTED_EDGE ( 'NONE', *, *, #7520, .T. ) ;
#9641=FACE_OUTER_BOUND ( 'NONE', #13742, .T. ) ;
#9646=CARTESIAN_POINT ( 'NONE',  ( 73.09088021254186174, 1.387778780781445676E-14, -19.99999999999999645 ) ) ;
#9654=CARTESIAN_POINT ( 'NONE',  ( -77.83224521979003896, 0.3113578409232161670, 4.597830265575576725 ) ) ;
#9658=EDGE_CURVE ( 'NONE', #3705, #5412, #3614, .T. ) ;
#9706=DIRECTION ( 'NONE',  ( 1.000000000000000000, 8.260059303211164661E-14, 0.000000000000000000 ) ) ;
#9719=AXIS2_PLACEMENT_3D ( 'NONE', #5754, #8309, #12836 ) ;
#9722=CARTESIAN_POINT ( 'NONE',  ( -170.4538399828638831, 32.22998840342273041, 4.764204982952881196 ) ) ;
#9730=LINE ( 'NONE', #13867, #5365 ) ;
#9757=DIRECTION ( 'NONE',  ( 1.000000000000000000, 0.000000000000000000, -2.478176394252581634E-16 ) ) ;
#9761=CARTESIAN_POINT ( 'NONE',  ( 73.09088021254186174, 1.387778780781445676E-14, 110.7545852194966045 ) ) ;
#9780=DIRECTION ( 'NONE',  ( 0.9201637183752249260, 0.3915338189555018777, 0.000000000000000000 ) ) ;
#9796=EDGE_LOOP ( 'NONE', ( #11375, #5134, #1883, #10825, #11294 ) ) ;
#9798=CIRCLE ( 'NONE', #14642, 145.0000000000000284 ) ;
#9805=CARTESIAN_POINT ( 'NONE',  ( -71.57226172492416083, 45.66900446655741774, 3.728993592375226207 ) ) ;
#9806=EDGE_CURVE ( 'NONE', #13271, #3138, #17321, .T. ) ;
#9845=DIRECTION ( 'NONE',  ( 0.1856185419698759831, -0.9826218788918641422, 0.000000000000000000 ) ) ;
#9851=CARTESIAN_POINT ( 'NONE',  ( 73.09088021254186174, 1.387778780781445676E-14, 25.00000000000000000 ) ) ;
#9863=VECTOR ( 'NONE', #6772, 1000.000000000000114 ) ;
#9865=FILL_AREA_STYLE_COLOUR ( '', #8866 ) ;
#9881=CARTESIAN_POINT ( 'NONE',  ( -59.79999999999999716, 0.000000000000000000, -25.00000000000000000 ) ) ;
#9897=DIRECTION ( 'NONE',  ( 0.000000000000000000, 0.000000000000000000, 1.000000000000000000 ) ) ;
#9905=DIRECTION ( 'NONE',  ( -0.000000000000000000, -0.000000000000000000, -1.000000000000000000 ) ) ;
#9909=VECTOR ( 'NONE', #6823, 1000.000000000000000 ) ;
#9912=ORIENTED_EDGE ( 'NONE', *, *, #12791, .T. ) ;
#9917=CARTESIAN_POINT ( 'NONE',  ( -77.24751462517671996, -0.7168438680194959556, 5.646068113733807792 ) ) ;
#9920=ORIENTED_EDGE ( 'NONE', *, *, #14373, .T. ) ;
#9927=CARTESIAN_POINT ( 'NONE',  ( -349.6046375497077179, 10.42115585936044830, 9.951701414186830458E-16 ) ) ;
#9934=DIRECTION ( 'NONE',  ( 0.000000000000000000, 0.000000000000000000, 1.000000000000000000 ) ) ;
#9954=CARTESIAN_POINT ( 'NONE',  ( -78.67338996650589422, 1.237145499066719001, -3.655658421838791750 ) ) ;
#9957=AXIS2_PLACEMENT_3D ( 'NONE', #13066, #10063, #11566 ) ;
#9977=DIRECTION ( 'NONE',  ( 0.9539392014169452150, -0.3000000000000013212, 0.000000000000000000 ) ) ;
#9989=FACE_BOUND ( 'NONE', #3062, .T. ) ;
#10037=EDGE_CURVE ( 'NONE', #18388, #411, #12105, .T. ) ;
#10039=EDGE_LOOP ( 'NONE', ( #13703, #276, #12942, #16328, #7953, #11272 ) ) ;
#10052=CARTESIAN_POINT ( 'NONE',  ( -79.05438463828195950, 1.499069270643396345, -3.389939594122236333 ) ) ;
#10056=( GEOMETRIC_REPRESENTATION_CONTEXT ( 3 ) GLOBAL_UNCERTAINTY_ASSIGNED_CONTEXT ( ( #16130 ) ) GLOBAL_UNIT_ASSIGNED_CONTEXT ( ( #9497, #10988, #109 ) ) REPRESENTATION_CONTEXT ( 'NONE', 'WORKASPACE' ) );
#10063=DIRECTION ( 'NONE',  ( -0.000000000000000000, -0.000000000000000000, -1.000000000000000000 ) ) ;
#10071=ORIENTED_EDGE ( 'NONE', *, *, #6271, .F. ) ;
#10080=ADVANCED_FACE ( 'NONE', ( #9277 ), #6463, .F. ) ;
#10081=CARTESIAN_POINT ( 'NONE',  ( -70.00000000000001421, 44.99999999999997868, -7.169095027853613189 ) ) ;
#10083=VERTEX_POINT ( 'NONE', #14967 ) ;
#10096=LINE ( 'NONE', #17423, #607 ) ;
#10126=ORIENTED_EDGE ( 'NONE', *, *, #16699, .T. ) ;
#10152=ORIENTED_EDGE ( 'NONE', *, *, #13875, .F. ) ;
#10155=ORIENTED_EDGE ( 'NONE', *, *, #5692, .F. ) ;
#10156=VECTOR ( 'NONE', #14983, 1000.000000000000000 ) ;
#10162=CARTESIAN_POINT ( 'NONE',  ( -174.8823813673296286, 55.30280195509305230, 5.132545408516865137 ) ) ;
#10163=DIRECTION ( 'NONE',  ( -1.000000000000000000, 0.000000000000000000, 0.000000000000000000 ) ) ;
#10170=AXIS2_PLACEMENT_3D ( 'NONE', #15426, #2446, #4029 ) ;
#10204=DIRECTION ( 'NONE',  ( -1.000000000000000000, 0.000000000000000000, 0.000000000000000000 ) ) ;
#10222=CARTESIAN_POINT ( 'NONE',  ( 2.200000000000000178, 2.694222958124177006E-16, 25.00000000000000000 ) ) ;
#10230=AXIS2_PLACEMENT_3D ( 'NONE', #8047, #9379, #479 ) ;
#10260=ORIENTED_EDGE ( 'NONE', *, *, #10990, .F. ) ;
#10262=CARTESIAN_POINT ( 'NONE',  ( -174.3165826136136332, 55.97625804580273012, 3.566331213966862368 ) ) ;
#10263=CYLINDRICAL_SURFACE ( 'NONE', #11761, 2.200000000000000622 ) ;
#10264=CARTESIAN_POINT ( 'NONE',  ( -174.8433004229789844, 55.46678263321123126, -4.764204982952879419 ) ) ;
#10268=CYLINDRICAL_SURFACE ( 'NONE', #2970, 2.200000000000000178 ) ;
#10277=EDGE_CURVE ( 'NONE', #7186, #14747, #3010, .T. ) ;
#10281=CARTESIAN_POINT ( 'NONE',  ( -69.99999999999998579, -45.00000000000000711, -19.99999999999999645 ) ) ;
#10291=VERTEX_POINT ( 'NONE', #10306 ) ;
#10292=DIRECTION ( 'NONE',  ( 2.671473304378624222E-16, 0.000000000000000000, 1.000000000000000000 ) ) ;
#10293=ORIENTED_EDGE ( 'NONE', *, *, #4439, .T. ) ;
#10301=DIRECTION ( 'NONE',  ( 1.000000000000000000, 0.000000000000000000, 0.000000000000000000 ) ) ;
#10305=DIRECTION ( 'NONE',  ( -1.000000000000000000, 0.000000000000000000, 0.000000000000000000 ) ) ;
#10306=CARTESIAN_POINT ( 'NONE',  ( -76.88766983611584749, -2.536636612185957595, 7.500000000000000000 ) ) ;
#10337=EDGE_LOOP ( 'NONE', ( #17008, #2827, #5773, #11985, #8335 ) ) ;
#10354=DIRECTION ( 'NONE',  ( -0.000000000000000000, -0.000000000000000000, -1.000000000000000000 ) ) ;
#10363=CARTESIAN_POINT ( 'NONE',  ( -172.7326993491721225, 43.83249341393818810, 9.951701414186830458E-16 ) ) ;
#10366=DIRECTION ( 'NONE',  ( -0.000000000000000000, -0.000000000000000000, -1.000000000000000000 ) ) ;
#10370=PLANE ( 'NONE',  #7863 ) ;
#10377=DIRECTION ( 'NONE',  ( -0.9826218788918641422, -0.1856185419698762606, 0.000000000000000000 ) ) ;
#10390=ORIENTED_EDGE ( 'NONE', *, *, #13342, .F. ) ;
#10392=CARTESIAN_POINT ( 'NONE',  ( -172.7326993491721225, 43.83249341393818810, 9.951701414186830458E-16 ) ) ;
#10411=CARTESIAN_POINT ( 'NONE',  ( -76.89338248673432474, -2.351275769351085732, -7.311503873159917788 ) ) ;
#10414=EDGE_CURVE ( 'NONE', #4333, #6623, #14601, .T. ) ;
#10418=CARTESIAN_POINT ( 'NONE',  ( 73.09088021254186174, 1.387778780781445676E-14, 19.99999999999997513 ) ) ;
#10427=LINE ( 'NONE', #3314, #10156 ) ;
#10446=DIRECTION ( 'NONE',  ( 0.1856185419698760941, -0.9826218788918640312, 0.000000000000000000 ) ) ;
#10448=ADVANCED_BREP_SHAPE_REPRESENTATION ( '', ( #8769, #18772 ), #18155 ) ;
#10464=DIRECTION ( 'NONE',  ( 1.000000000000000000, 0.000000000000000000, 0.000000000000000000 ) ) ;
#10465=EDGE_CURVE ( 'NONE', #6411, #16662, #12464, .T. ) ;
#10473=EDGE_CURVE ( 'NONE', #7569, #2144, #4593, .T. ) ;
#10507=ORIENTED_EDGE ( 'NONE', *, *, #4474, .T. ) ;
#10526=EDGE_CURVE ( 'NONE', #9141, #4403, #13784, .T. ) ;
#10535=FACE_OUTER_BOUND ( 'NONE', #16206, .T. ) ;
#10540=MECHANICAL_DESIGN_GEOMETRIC_PRESENTATION_REPRESENTATION('',(#5726),#4484);
#10541=B_SPLINE_CURVE_WITH_KNOTS ( 'NONE', 3,
 ( #10052, #9954, #8728, #15841, #1629, #15749, #2770, #8556, #7232, #14513, #1539, #13084, #11726, #10411, #4724, #3295 ),
 .UNSPECIFIED., .F., .F.,
 ( 4, 2, 2, 2, 2, 2, 2, 4 ),
 ( 0.000000000000000000, 0.001565668136846128924, 0.002348502205269182869, 0.003131336273692236598, 0.004697004410538344922, 0.005479838478961394747, 0.005871255513172918793, 0.006262672547384443705 ),
 .UNSPECIFIED. ) ;
#10544=VERTEX_POINT ( 'NONE', #2530 ) ;
#10548=FACE_OUTER_BOUND ( 'NONE', #3846, .T. ) ;
#10586=PRODUCT_DEFINITION_SHAPE ( 'NONE', 'NONE',  #16949 ) ;
#10601=ORIENTED_EDGE ( 'NONE', *, *, #11151, .F. ) ;
#10605=DIRECTION ( 'NONE',  ( -0.9826218788918642533, -0.1856185419698762884, 0.000000000000000000 ) ) ;
#10611=CARTESIAN_POINT ( 'NONE',  ( -70.00000000000000000, 44.99999999999999289, 25.00000000000000000 ) ) ;
#10624=ORIENTED_EDGE ( 'NONE', *, *, #9156, .F. ) ;
#10635=VERTEX_POINT ( 'NONE', #1130 ) ;
#10645=CARTESIAN_POINT ( 'NONE',  ( -74.01655979591544110, 46.70906433774060673, -2.532234642382003909 ) ) ;
#10671=CARTESIAN_POINT ( 'NONE',  ( -69.99999999999998579, -45.00000000000000711, -19.99999999999999645 ) ) ;
#10675=VECTOR ( 'NONE', #16489, 1000.000000000000000 ) ;
#10689=DIRECTION ( 'NONE',  ( 0.9201637183752249260, -0.3915338189555017667, 0.000000000000000000 ) ) ;
#10697=CARTESIAN_POINT ( 'NONE',  ( -346.6567719130321166, 10.97801148527007697, 9.951701414186830458E-16 ) ) ;
#10701=DIRECTION ( 'NONE',  ( 1.000000000000000000, 0.000000000000000000, -2.631994239413086031E-16 ) ) ;
#10716=DIRECTION ( 'NONE',  ( -0.9826218788918642533, -0.1856185419698762884, 0.000000000000000000 ) ) ;
#10721=DIRECTION ( 'NONE',  ( 0.000000000000000000, 0.000000000000000000, 1.000000000000000000 ) ) ;
#10750=CYLINDRICAL_SURFACE ( 'NONE', #4338, 3.000000000000001776 ) ;
#10760=CARTESIAN_POINT ( 'NONE',  ( -62.00000000000000000, 0.000000000000000000, -25.00000000000000000 ) ) ;
#10773=AXIS2_PLACEMENT_3D ( 'NONE', #6260, #10605, #3197 ) ;
#10783=AXIS2_PLACEMENT_3D ( 'NONE', #10760, #6452, #751 ) ;
#10803=LINE ( 'NONE', #7899, #14822 ) ;
#10807=DIRECTION ( 'NONE',  ( -1.000000000000000000, 0.000000000000000000, 0.000000000000000000 ) ) ;
#10815=CARTESIAN_POINT ( 'NONE',  ( -172.4933171327469097, 56.54760101112823634, -2.520603730400377884 ) ) ;
#10825=ORIENTED_EDGE ( 'NONE', *, *, #2005, .F. ) ;
#10837=VERTEX_POINT ( 'NONE', #7822 ) ;
#10856=DIRECTION ( 'NONE',  ( -0.000000000000000000, -0.000000000000000000, -1.000000000000000000 ) ) ;
#10902=LINE ( 'NONE', #9588, #4538 ) ;
#10904=FACE_OUTER_BOUND ( 'NONE', #10039, .T. ) ;
#10912=CARTESIAN_POINT ( 'NONE',  ( -170.2279335768367048, 32.06947484904029011, -4.224609204322613998 ) ) ;
#10919=CARTESIAN_POINT ( 'NONE',  ( -69.99999999999998579, -45.00000000000000711, 20.00000000000001776 ) ) ;
#10927=PLANE ( 'NONE',  #6038 ) ;
#10929=VECTOR ( 'NONE', #8659, 1000.000000000000000 ) ;
#10955=DIRECTION ( 'NONE',  ( -0.000000000000000000, -0.000000000000000000, -1.000000000000000000 ) ) ;
#10964=ADVANCED_FACE ( 'NONE', ( #530, #9431, #9615 ), #10927, .F. ) ;
#10965=DIRECTION ( 'NONE',  ( 0.1856185419698762329, -0.9826218788918640312, 0.000000000000000000 ) ) ;
#10978=AXIS2_PLACEMENT_3D ( 'NONE', #9255, #14944, #10305 ) ;
#10988=( NAMED_UNIT ( * ) PLANE_ANGLE_UNIT ( ) SI_UNIT ( $, .RADIAN. ) );
#10990=EDGE_CURVE ( 'NONE', #7954, #15891, #5632, .T. ) ;
#10995=DIRECTION ( 'NONE',  ( 0.9201637183752248150, -0.3915338189555022108, 0.000000000000000000 ) ) ;
#11004=ORIENTED_EDGE ( 'NONE', *, *, #9806, .F. ) ;
#11005=LINE ( 'NONE', #10919, #12733 ) ;
#11011=CARTESIAN_POINT ( 'NONE',  ( -70.23909404122630917, 45.10173559463541437, 5.879686486593318939 ) ) ;
#11012=CARTESIAN_POINT ( 'NONE',  ( -70.00000000000000000, 44.99999999999999289, 25.00000000000000000 ) ) ;
#11020=VERTEX_POINT ( 'NONE', #18479 ) ;
#11037=SHAPE_REPRESENTATION_RELATIONSHIP ( 'NONE' , 'NONE' ,  #5397, #10448 ) ;
#11039=B_SPLINE_CURVE_WITH_KNOTS ( 'NONE', 3,
 ( #4235, #5291, #2626, #8413, #9917, #15815, #14387, #9654, #4128, #15523, #14095, #18616 ),
 .UNSPECIFIED., .F., .F.,
 ( 4, 2, 2, 2, 2, 4 ),
 ( -1.414213904430124076E-05, 0.001573093992944416377, 0.003160330124933133974, 0.003953948190927493098, 0.004747566256921851788, 0.006334802388910591719 ),
 .UNSPECIFIED. ) ;
#11057=EDGE_LOOP ( 'NONE', ( #13409, #6931, #1600, #13404 ) ) ;
#11064=DIRECTION ( 'NONE',  ( -0.9201637183752250371, 0.3915338189555017112, -0.000000000000000000 ) ) ;
#11086=DIRECTION ( 'NONE',  ( -0.9539392014169441047, -0.3000000000000045963, 0.000000000000000000 ) ) ;
#11094=EDGE_CURVE ( 'NONE', #3775, #8040, #15388, .T. ) ;
#11103=ORIENTED_EDGE ( 'NONE', *, *, #13132, .F. ) ;
#11124=VECTOR ( 'NONE', #844, 1000.000000000000000 ) ;
#11145=CARTESIAN_POINT ( 'NONE',  ( -71.90911978745813826, 1.387778780781445676E-14, 110.7545852194966045 ) ) ;
#11146=LINE ( 'NONE', #18228, #17856 ) ;
#11151=EDGE_CURVE ( 'NONE', #10291, #15850, #18580, .T. ) ;
#11160=CARTESIAN_POINT ( 'NONE',  ( -168.4538323585589694, 31.95594125380572947, -2.500000000000000000 ) ) ;
#11169=AXIS2_PLACEMENT_3D ( 'NONE', #14112, #7043, #15623 ) ;
#11178=CARTESIAN_POINT ( 'NONE',  ( -69.99999999999998579, -45.00000000000000711, 25.00000000000000000 ) ) ;
#11195=EDGE_LOOP ( 'NONE', ( #7497, #13351, #16040 ) ) ;
#11210=DIRECTION ( 'NONE',  ( -0.000000000000000000, -0.000000000000000000, -1.000000000000000000 ) ) ;
#11225=ORIENTED_EDGE ( 'NONE', *, *, #8870, .F. ) ;
#11238=SURFACE_STYLE_FILL_AREA ( #18106 ) ;
#11242=CARTESIAN_POINT ( 'NONE',  ( -172.0951522251743029, 56.61964399677355431, -2.500000000000000000 ) ) ;
#11250=VERTEX_POINT ( 'NONE', #9477 ) ;
#11251=ORIENTED_EDGE ( 'NONE', *, *, #13888, .F. ) ;
#11259=CARTESIAN_POINT ( 'NONE',  ( -81.87192997736543987, 3.395211045985502274, -2.500000000000000000 ) ) ;
#11262=EDGE_LOOP ( 'NONE', ( #3087, #3362, #18056, #8572, #12228, #16902, #5176 ) ) ;
#11263=FACE_OUTER_BOUND ( 'NONE', #6822, .T. ) ;
#11266=CARTESIAN_POINT ( 'NONE',  ( -76.90911978745816668, -45.00000000000000711, -20.00000000000000000 ) ) ;
#11271=MECHANICAL_DESIGN_GEOMETRIC_PRESENTATION_REPRESENTATION('',(#18286),#10056);
#11272=ORIENTED_EDGE ( 'NONE', *, *, #10990, .T. ) ;
#11294=ORIENTED_EDGE ( 'NONE', *, *, #15551, .F. ) ;
#11317=DIRECTION ( 'NONE',  ( -1.000000000000000000, 0.000000000000000000, 0.000000000000000000 ) ) ;
#11330=ADVANCED_FACE ( 'NONE', ( #13439 ), #2082, .T. ) ;
#11349=B_SPLINE_CURVE_WITH_KNOTS ( 'NONE', 3,
 ( #11259, #5400, #2260, #18133, #2465, #18244 ),
 .UNSPECIFIED., .F., .F.,
 ( 4, 2, 4 ),
 ( 3.705370968959021185E-18, 0.001760439274641287504, 0.003520878549282571539 ),
 .UNSPECIFIED. ) ;
#11359=ORIENTED_EDGE ( 'NONE', *, *, #7293, .F. ) ;
#11375=ORIENTED_EDGE ( 'NONE', *, *, #18358, .T. ) ;
#11383=FACE_OUTER_BOUND ( 'NONE', #6826, .T. ) ;
#11386=ADVANCED_FACE ( 'NONE', ( #17950 ), #6934, .T. ) ;
#11394=ORIENTED_EDGE ( 'NONE', *, *, #17782, .F. ) ;
#11403=AXIS2_PLACEMENT_3D ( 'NONE', #13622, #12388, #16577 ) ;
#11408=CARTESIAN_POINT ( 'NONE',  ( -70.00000000000000000, 44.99999999999999289, 2.500000000000000000 ) ) ;
#11409=ADVANCED_FACE ( 'NONE', ( #16590 ), #7959, .F. ) ;
#11419=ORIENTED_EDGE ( 'NONE', *, *, #11094, .T. ) ;
#11442=DIRECTION ( 'NONE',  ( 3.816390434826605238E-17, 0.000000000000000000, -1.000000000000000000 ) ) ;
#11475=ORIENTED_EDGE ( 'NONE', *, *, #5692, .T. ) ;
#11484=CARTESIAN_POINT ( 'NONE',  ( -174.8836385705398300, 55.21907105134628324, 5.316095106350546828 ) ) ;
#11519=EDGE_CURVE ( 'NONE', #16333, #411, #4255, .T. ) ;
#11530=DIRECTION ( 'NONE',  ( -0.000000000000000000, -0.000000000000000000, -1.000000000000000000 ) ) ;
#11538=CIRCLE ( 'NONE', #13976, 150.0000000000000284 ) ;
#11561=VECTOR ( 'NONE', #13754, 1000.000000000000000 ) ;
#11566=DIRECTION ( 'NONE',  ( -1.000000000000000000, 0.000000000000000000, 0.000000000000000000 ) ) ;
#11579=EDGE_CURVE ( 'NONE', #518, #7954, #3868, .T. ) ;
#11584=CARTESIAN_POINT ( 'NONE',  ( -174.8436531212914815, 55.46571492669004755, 4.766626691765358359 ) ) ;
#11587=B_SPLINE_CURVE_WITH_KNOTS ( 'NONE', 3,
 ( #16888, #15246, #11160, #14105 ),
 .UNSPECIFIED., .F., .F.,
 ( 4, 4 ),
 ( 0.000000000000000000, 0.003000475340473835600 ),
 .UNSPECIFIED. ) ;
#11597=VERTEX_POINT ( 'NONE', #15830 ) ;
#11660=CARTESIAN_POINT ( 'NONE',  ( -170.4124675745486570, 31.54971992778987655, 2.500000000000000000 ) ) ;
#11700=AXIS2_PLACEMENT_3D ( 'NONE', #4941, #1936, #17893 ) ;
#11705=DIRECTION ( 'NONE',  ( -0.9201637183752249260, -0.3915338189555018777, 0.000000000000000000 ) ) ;
#11722=VERTEX_POINT ( 'NONE', #13418 ) ;
#11726=CARTESIAN_POINT ( 'NONE',  ( -76.90684458043445204, -2.166085715380211774, -7.123062958295337310 ) ) ;
#11739=ORIENTED_EDGE ( 'NONE', *, *, #2372, .F. ) ;
#11756=CARTESIAN_POINT ( 'NONE',  ( -72.30733464426469936, 45.98178131438659477, -3.159861247684372820 ) ) ;
#11761=AXIS2_PLACEMENT_3D ( 'NONE', #6004, #1732, #7626 ) ;
#11768=AXIS2_PLACEMENT_3D ( 'NONE', #12992, #2853, #18653 ) ;
#11779=AXIS2_PLACEMENT_3D ( 'NONE', #9761, #6922, #15527 ) ;
#11782=CARTESIAN_POINT ( 'NONE',  ( 0.000000000000000000, 0.000000000000000000, 25.00000000000000000 ) ) ;
#11783=ORIENTED_EDGE ( 'NONE', *, *, #6849, .F. ) ;
#11811=VERTEX_POINT ( 'NONE', #7671 ) ;
#11836=CARTESIAN_POINT ( 'NONE',  ( -64.20000000000000284, 2.694222958124175527E-16, -25.00000000000000000 ) ) ;
#11843=CARTESIAN_POINT ( 'NONE',  ( -175.0529311237955881, 56.11526690008648899, -2.500000000000065725 ) ) ;
#11844=ORIENTED_EDGE ( 'NONE', *, *, #7288, .T. ) ;
#11867=ORIENTED_EDGE ( 'NONE', *, *, #4266, .T. ) ;
#11870=CARTESIAN_POINT ( 'NONE',  ( -65.23030399291528170, -43.49999999999991473, 110.7545852194966045 ) ) ;
#11873=EDGE_CURVE ( 'NONE', #18049, #13271, #15714, .T. ) ;
#11908=DIRECTION ( 'NONE',  ( -0.9826218788918642533, -0.1856185419698762884, 0.000000000000000000 ) ) ;
#11945=DIRECTION ( 'NONE',  ( -1.000000000000000000, 0.000000000000000000, 0.000000000000000000 ) ) ;
#11976=ORIENTED_EDGE ( 'NONE', *, *, #5595, .T. ) ;
#11980=CARTESIAN_POINT ( 'NONE',  ( -176.1167811578620501, -139.6880237571007513, 2.500000000000000000 ) ) ;
#11981=FACE_OUTER_BOUND ( 'NONE', #12446, .T. ) ;
#11983=CYLINDRICAL_SURFACE ( 'NONE', #9957, 149.4844750268700864 ) ;
#11985=ORIENTED_EDGE ( 'NONE', *, *, #10037, .T. ) ;
#12019=ORIENTED_EDGE ( 'NONE', *, *, #12410, .F. ) ;
#12057=VECTOR ( 'NONE', #7047, 1000.000000000000000 ) ;
#12078=CARTESIAN_POINT ( 'NONE',  ( 0.000000000000000000, 0.000000000000000000, -25.00000000000000000 ) ) ;
#12091=CIRCLE ( 'NONE', #6993, 150.0000000000000284 ) ;
#12092=LINE ( 'NONE', #3663, #4753 ) ;
#12105=LINE ( 'NONE', #10611, #987 ) ;
#12114=CARTESIAN_POINT ( 'NONE',  ( -69.99999999999998579, -45.00000000000000711, -25.00000000000000000 ) ) ;
#12131=CARTESIAN_POINT ( 'NONE',  ( 73.09088021254186174, 1.387778780781445676E-14, -19.99999999999999645 ) ) ;
#12133=CARTESIAN_POINT ( 'NONE',  ( 5.481473465377026066, -12.88229205725314586, 20.00000000000000000 ) ) ;
#12134=DIRECTION ( 'NONE',  ( -0.000000000000000000, -0.000000000000000000, -1.000000000000000000 ) ) ;
#12152=CYLINDRICAL_SURFACE ( 'NONE', #3963, 5.000000000000004441 ) ;
#12195=EDGE_CURVE ( 'NONE', #9141, #4403, #1227, .T. ) ;
#12199=DIRECTION ( 'NONE',  ( 0.1856185419698762884, -0.9826218788918641422, 0.000000000000000000 ) ) ;
#12219=ORIENTED_EDGE ( 'NONE', *, *, #8292, .F. ) ;
#12228=ORIENTED_EDGE ( 'NONE', *, *, #17775, .F. ) ;
#12236=CARTESIAN_POINT ( 'NONE',  ( -174.4265963546509965, 55.91158385207030790, -3.719291248522901050 ) ) ;
#12244=CARTESIAN_POINT ( 'NONE',  ( -72.57741747767370555, 46.09670278008585598, 3.004020071001521686 ) ) ;
#12252=ORIENTED_EDGE ( 'NONE', *, *, #955, .F. ) ;
#12311=PRESENTATION_STYLE_ASSIGNMENT (( #6567 ) ) ;
#12327=CARTESIAN_POINT ( 'NONE',  ( -169.3393727017007677, 31.92299471093763685, -3.150553392547038367 ) ) ;
#12338=CARTESIAN_POINT ( 'NONE',  ( -71.14534172961498371, 45.48734807996677176, 4.189415517288649582 ) ) ;
#12341=B_SPLINE_CURVE_WITH_KNOTS ( 'NONE', 3,
 ( #8700, #2740, #15611, #12949 ),
 .UNSPECIFIED., .F., .F.,
 ( 4, 4 ),
 ( 0.000000000000000000, 0.003000475340473846009 ),
 .UNSPECIFIED. ) ;
#12369=AXIS2_PLACEMENT_3D ( 'NONE', #15628, #1165, #18446 ) ;
#12388=DIRECTION ( 'NONE',  ( 0.000000000000000000, 0.000000000000000000, 1.000000000000000000 ) ) ;
#12402=CARTESIAN_POINT ( 'NONE',  ( -172.7326993491721225, 43.83249341393818810, 9.951701414186830458E-16 ) ) ;
#12409=EDGE_LOOP ( 'NONE', ( #3687, #5409, #4943 ) ) ;
#12410=EDGE_CURVE ( 'NONE', #113, #11250, #8481, .T. ) ;
#12412=ORIENTED_EDGE ( 'NONE', *, *, #11151, .T. ) ;
#12416=CARTESIAN_POINT ( 'NONE',  ( -76.90911978745816668, 1.387778780781445676E-14, 25.00000000000000000 ) ) ;
#12436=CARTESIAN_POINT ( 'NONE',  ( -167.8744510809501378, 32.07610638047782459, -2.499999999999995559 ) ) ;
#12446=EDGE_LOOP ( 'NONE', ( #11251, #11739, #1144, #11225, #797, #9505 ) ) ;
#12457=VECTOR ( 'NONE', #18555, 1000.000000000000227 ) ;
#12460=VERTEX_POINT ( 'NONE', #11660 ) ;
#12464=CIRCLE ( 'NONE', #12763, 13.99999999999999822 ) ;
#12484=EDGE_CURVE ( 'NONE', #4403, #17089, #13179, .T. ) ;
#12524=CARTESIAN_POINT ( 'NONE',  ( -170.3900270404893718, 32.17034444718320430, -4.582591203971097649 ) ) ;
#12527=CARTESIAN_POINT ( 'NONE',  ( -64.20000000000000284, 2.694222958124180951E-16, -25.00000000000000000 ) ) ;
#12529=CARTESIAN_POINT ( 'NONE',  ( -168.8245792648350516, 31.94895759036034377, 2.821239268406344536 ) ) ;
#12535=AXIS2_PLACEMENT_3D ( 'NONE', #13446, #3400, #14789 ) ;
#12549=AXIS2_PLACEMENT_3D ( 'NONE', #7455, #10377, #13216 ) ;
#12560=ORIENTED_EDGE ( 'NONE', *, *, #18408, .T. ) ;
#12571=CARTESIAN_POINT ( 'NONE',  ( -74.62210677719829732, 46.96672731380024146, 2.500000000000000000 ) ) ;
#12585=CYLINDRICAL_SURFACE ( 'NONE', #12369, 2.200000000000000622 ) ;
#12620=DIRECTION ( 'NONE',  ( 1.000000000000000000, 0.000000000000000000, -0.000000000000000000 ) ) ;
#12634=AXIS2_PLACEMENT_3D ( 'NONE', #4587, #10721, #9223 ) ;
#12640=ADVANCED_FACE ( 'NONE', ( #4934 ), #17780, .F. ) ;
#12661=AXIS2_PLACEMENT_3D ( 'NONE', #18365, #3707, #10807 ) ;
#12680=AXIS2_PLACEMENT_3D ( 'NONE', #2597, #6988, #5550 ) ;
#12682=APPLICATION_CONTEXT ( 'automotive_design' ) ;
#12683=FACE_OUTER_BOUND ( 'NONE', #11057, .T. ) ;
#12684=LINE ( 'NONE', #17088, #7544 ) ;
#12691=CIRCLE ( 'NONE', #6986, 12.83663829214476948 ) ;
#12700=LINE ( 'NONE', #1084, #12457 ) ;
#12706=AXIS2_PLACEMENT_3D ( 'NONE', #15315, #15134, #2153 ) ;
#12717=DIRECTION ( 'NONE',  ( 0.9201637183752249260, 0.3915338189555018777, -2.458192809297183803E-16 ) ) ;
#12733=VECTOR ( 'NONE', #12717, 1000.000000000000114 ) ;
#12734=DIRECTION ( 'NONE',  ( 0.1856185419698760941, -0.9826218788918640312, 0.000000000000000000 ) ) ;
#12735=ORIENTED_EDGE ( 'NONE', *, *, #17754, .T. ) ;
#12741=EDGE_CURVE ( 'NONE', #13951, #11811, #10902, .T. ) ;
#12750=CARTESIAN_POINT ( 'NONE',  ( -69.99999999999998579, -45.00000000000000711, 110.7545852194966045 ) ) ;
#12761=DIRECTION ( 'NONE',  ( 3.816390434826605238E-17, 0.000000000000000000, -1.000000000000000000 ) ) ;
#12763=AXIS2_PLACEMENT_3D ( 'NONE', #4702, #7669, #2156 ) ;
#12769=ADVANCED_FACE ( 'NONE', ( #2285 ), #8279, .F. ) ;
#12791=EDGE_CURVE ( 'NONE', #15850, #14394, #12091, .T. ) ;
#12811=FACE_OUTER_BOUND ( 'NONE', #17411, .T. ) ;
#12815=VERTEX_POINT ( 'NONE', #8177 ) ;
#12821=CARTESIAN_POINT ( 'NONE',  ( -62.00000000000000000, 0.000000000000000000, -25.00000000000000000 ) ) ;
#12822=CARTESIAN_POINT ( 'NONE',  ( -59.79999999999999716, 0.000000000000000000, -20.00000000000000000 ) ) ;
#12827=CARTESIAN_POINT ( 'NONE',  ( -174.6164565666191777, 55.77096170148206511, 4.052748550462854205 ) ) ;
#12830=CARTESIAN_POINT ( 'NONE',  ( -172.7326993491721225, 43.83249341393818810, 9.951701414186830458E-16 ) ) ;
#12831=ORIENTED_EDGE ( 'NONE', *, *, #3787, .F. ) ;
#12832=EDGE_LOOP ( 'NONE', ( #2923, #12019, #12914, #17396 ) ) ;
#12836=DIRECTION ( 'NONE',  ( 1.000000000000000000, 0.000000000000000000, 0.000000000000000000 ) ) ;
#12871=DIRECTION ( 'NONE',  ( 0.9201637183752250371, -0.3915338189555017667, 3.511704013281690619E-17 ) ) ;
#12875=LINE ( 'NONE', #1262, #12057 ) ;
#12877=ORIENTED_EDGE ( 'NONE', *, *, #13082, .T. ) ;
#12879=CARTESIAN_POINT ( 'NONE',  ( -172.0951522251743029, 56.61964399677356141, 2.500000000000000000 ) ) ;
#12903=VECTOR ( 'NONE', #17452, 1000.000000000000114 ) ;
#12911=CARTESIAN_POINT ( 'NONE',  ( -173.4308285199811905, 56.32218110407216471, 2.822349119005441054 ) ) ;
#12914=ORIENTED_EDGE ( 'NONE', *, *, #8979, .T. ) ;
#12915=ORIENTED_EDGE ( 'NONE', *, *, #13738, .T. ) ;
#12928=FACE_OUTER_BOUND ( 'NONE', #6158, .T. ) ;
#12937=EDGE_LOOP ( 'NONE', ( #10624, #4954, #2212, #16761, #16942, #9012 ) ) ;
#12942=ORIENTED_EDGE ( 'NONE', *, *, #14636, .T. ) ;
#12949=CARTESIAN_POINT ( 'NONE',  ( -170.4124675745486570, 31.54971992778987655, 2.500000000000000000 ) ) ;
#12955=CARTESIAN_POINT ( 'NONE',  ( -65.23030399291525327, 43.49999999999997868, 110.7545852194966045 ) ) ;
#12980=DIRECTION ( 'NONE',  ( -2.671473304378624222E-16, -0.000000000000000000, -1.000000000000000000 ) ) ;
#12990=AXIS2_PLACEMENT_3D ( 'NONE', #7279, #4500, #13210 ) ;
#12992=CARTESIAN_POINT ( 'NONE',  ( -169.7848337124965212, 44.38934903984782210, -5.500000000000000000 ) ) ;
#12994=ORIENTED_EDGE ( 'NONE', *, *, #6488, .F. ) ;
#13021=ADVANCED_FACE ( 'NONE', ( #9206 ), #15068, .F. ) ;
#13033=VECTOR ( 'NONE', #10366, 1000.000000000000000 ) ;
#13047=VERTEX_POINT ( 'NONE', #11836 ) ;
#13051=CARTESIAN_POINT ( 'NONE',  ( -349.5448134615015761, 26.54870825572371018, 2.934543024899866731E-15 ) ) ;
#13053=AXIS2_PLACEMENT_3D ( 'NONE', #3326, #9130, #1923 ) ;
#13054=CYLINDRICAL_SURFACE ( 'NONE', #18635, 150.0000000000000284 ) ;
#13062=DIRECTION ( 'NONE',  ( -0.9792327305835186735, -0.2027393877714586679, 0.000000000000000000 ) ) ;
#13065=PLANE ( 'NONE',  #11169 ) ;
#13066=CARTESIAN_POINT ( 'NONE',  ( -137.7298645655810390, -88.63485219053825404, 2.500000000000000000 ) ) ;
#13082=EDGE_CURVE ( 'NONE', #4539, #15554, #16500, .T. ) ;
#13083=EDGE_CURVE ( 'NONE', #13047, #7914, #17574, .T. ) ;
#13084=CARTESIAN_POINT ( 'NONE',  ( -76.91617387511415416, -2.073484822433842911, -7.028799330061641371 ) ) ;
#13092=DIRECTION ( 'NONE',  ( -1.000000000000000000, 0.000000000000000000, 0.000000000000000000 ) ) ;
#13094=ORIENTED_EDGE ( 'NONE', *, *, #12195, .F. ) ;
#13099=CARTESIAN_POINT ( 'NONE',  ( -70.00000000000000000, 44.99999999999999289, 110.7545852194966045 ) ) ;
#13111=CARTESIAN_POINT ( 'NONE',  ( -137.7298645655810390, -88.63485219053825404, 2.500000000000000000 ) ) ;
#13132=EDGE_CURVE ( 'NONE', #10635, #4836, #15575, .T. ) ;
#13163=DIRECTION ( 'NONE',  ( 0.000000000000000000, 0.000000000000000000, 1.000000000000000000 ) ) ;
#13179=B_SPLINE_CURVE_WITH_KNOTS ( 'NONE', 3,
 ( #1299, #11484, #10162, #11584, #4390, #4482, #12827, #6003, #10262, #14544, #7165, #13188, #12911, #2868, #5739, #8667 ),
 .UNSPECIFIED., .F., .F.,
 ( 4, 2, 2, 2, 2, 2, 2, 4 ),
 ( 1.734723475976807094E-18, 0.0006035471611761495346, 0.001207094322352297334, 0.001810641483528445134, 0.002414188644704592934, 0.003017735805880740734, 0.003621282967056888534, 0.004828377289409252655 ),
 .UNSPECIFIED. ) ;
#13185=CIRCLE ( 'NONE', #15008, 150.0000000000000284 ) ;
#13186=CIRCLE ( 'NONE', #5008, 2.200000000000000178 ) ;
#13188=CARTESIAN_POINT ( 'NONE',  ( -173.6030297042496500, 56.26981074892695034, 2.921574671186270677 ) ) ;
#13189=CARTESIAN_POINT ( 'NONE',  ( -2.200000000000000178, 0.000000000000000000, 20.00000000000000000 ) ) ;
#13191=CARTESIAN_POINT ( 'NONE',  ( -174.8673125818257006, 55.13264502119463373, -5.500000000000001776 ) ) ;
#13192=LINE ( 'NONE', #5917, #13465 ) ;
#13205=VERTEX_POINT ( 'NONE', #11242 ) ;
#13210=DIRECTION ( 'NONE',  ( 1.000000000000000000, 0.000000000000000000, 0.000000000000000000 ) ) ;
#13216=DIRECTION ( 'NONE',  ( 0.1856185419698762329, -0.9826218788918640312, 0.000000000000000000 ) ) ;
#13219=ORIENTED_EDGE ( 'NONE', *, *, #4173, .T. ) ;
#13271=VERTEX_POINT ( 'NONE', #7017 ) ;
#13342=EDGE_CURVE ( 'NONE', #16721, #518, #15205, .T. ) ;
#13351=ORIENTED_EDGE ( 'NONE', *, *, #17803, .T. ) ;
#13391=CARTESIAN_POINT ( 'NONE',  ( 2.200000000000000178, 2.694222958124177006E-16, 20.00000000000000000 ) ) ;
#13404=ORIENTED_EDGE ( 'NONE', *, *, #7520, .F. ) ;
#13409=ORIENTED_EDGE ( 'NONE', *, *, #16765, .F. ) ;
#13412=AXIS2_PLACEMENT_3D ( 'NONE', #18217, #742, #6523 ) ;
#13418=CARTESIAN_POINT ( 'NONE',  ( -81.87192997736543987, 3.395211045985502274, -2.500000000000000000 ) ) ;
#13434=ORIENTED_EDGE ( 'NONE', *, *, #359, .T. ) ;
#13439=FACE_OUTER_BOUND ( 'NONE', #14220, .T. ) ;
#13446=CARTESIAN_POINT ( 'NONE',  ( -176.1167811578620501, -139.6880237571007513, 2.500000000000000000 ) ) ;
#13458=ADVANCED_FACE ( 'NONE', ( #1405 ), #2986, .F. ) ;
#13465=VECTOR ( 'NONE', #3148, 1000.000000000000114 ) ;
#13477=FACE_OUTER_BOUND ( 'NONE', #11195, .T. ) ;
#13481=AXIS2_PLACEMENT_3D ( 'NONE', #780, #18150, #9490 ) ;
#13490=ORIENTED_EDGE ( 'NONE', *, *, #10526, .T. ) ;
#13494=AXIS2_PLACEMENT_3D ( 'NONE', #11266, #11442, #15622 ) ;
#13510=AXIS2_PLACEMENT_3D ( 'NONE', #1681, #256, #6150 ) ;
#13523=LINE ( 'NONE', #16409, #15495 ) ;
#13525=LINE ( 'NONE', #574, #10675 ) ;
#13550=AXIS2_PLACEMENT_3D ( 'NONE', #10392, #4797, #18014 ) ;
#13585=DIRECTION ( 'NONE',  ( 0.1856185419698760941, -0.9826218788918640312, 0.000000000000000000 ) ) ;
#13587=CYLINDRICAL_SURFACE ( 'NONE', #18429, 2.200000000000000178 ) ;
#13594=ADVANCED_FACE ( 'NONE', ( #536 ), #16462, .T. ) ;
#13596=VECTOR ( 'NONE', #4170, 1000.000000000000000 ) ;
#13611=CARTESIAN_POINT ( 'NONE',  ( 0.000000000000000000, 0.000000000000000000, 0.000000000000000000 ) ) ;
#13622=CARTESIAN_POINT ( 'NONE',  ( 73.09088021254186174, 1.387778780781445676E-14, 25.00000000000000000 ) ) ;
#13627=ORIENTED_EDGE ( 'NONE', *, *, #14355, .T. ) ;
#13657=AXIS2_PLACEMENT_3D ( 'NONE', #7867, #3674, #15245 ) ;
#13664=ORIENTED_EDGE ( 'NONE', *, *, #6028, .T. ) ;
#13672=CARTESIAN_POINT ( 'NONE',  ( -170.1307959478061491, 32.02908766448062750, 4.051035741711875637 ) ) ;
#13673=CARTESIAN_POINT ( 'NONE',  ( -172.8790805967747133, 56.46496941305928630, -2.601363783521513540 ) ) ;
#13675=AXIS2_PLACEMENT_3D ( 'NONE', #3457, #17820, #9256 ) ;
#13696=FACE_OUTER_BOUND ( 'NONE', #14411, .T. ) ;
#13700=CARTESIAN_POINT ( 'NONE',  ( -70.00000000000000000, 44.99999999999999289, -2.500000000000000000 ) ) ;
#13703=ORIENTED_EDGE ( 'NONE', *, *, #5880, .T. ) ;
#13706=DIRECTION ( 'NONE',  ( 1.000000000000000000, 0.000000000000000000, 0.000000000000000000 ) ) ;
#13734=SURFACE_SIDE_STYLE ('',( #7978 ) ) ;
#13738=EDGE_CURVE ( 'NONE', #5191, #17705, #165, .T. ) ;
#13742=EDGE_LOOP ( 'NONE', ( #6090, #14413, #1008, #4635, #16354, #1719, #15097 ) ) ;
#13746=DIRECTION ( 'NONE',  ( -0.9201637183752250371, 0.3915338189555017667, 2.458192809297184296E-16 ) ) ;
#13752=ORIENTED_EDGE ( 'NONE', *, *, #17993, .F. ) ;
#13754=DIRECTION ( 'NONE',  ( -0.000000000000000000, -0.000000000000000000, 1.000000000000000000 ) ) ;
#13757=CARTESIAN_POINT ( 'NONE',  ( -167.6743523352497789, 32.11760736101219038, 2.500000000000000888 ) ) ;
#13758=CARTESIAN_POINT ( 'NONE',  ( -173.0699421713717925, 56.41947239034702477, -2.662644313562635201 ) ) ;
#13770=ADVANCED_FACE ( 'NONE', ( #4205, #9989, #7359 ), #17223, .F. ) ;
#13778=EDGE_LOOP ( 'NONE', ( #5995, #18148, #3637, #1720 ) ) ;
#13784=LINE ( 'NONE', #15419, #6740 ) ;
#13818=ORIENTED_EDGE ( 'NONE', *, *, #16610, .F. ) ;
#13820=CARTESIAN_POINT ( 'NONE',  ( -80.87641299911182102, 2.735640769738576505, 2.577396323571959691 ) ) ;
#13824=AXIS2_PLACEMENT_3D ( 'NONE', #18231, #8241, #15434 ) ;
#13849=CARTESIAN_POINT ( 'NONE',  ( -169.0061012838959584, 31.93472873824967806, -2.921574671186277339 ) ) ;
#13856=DIRECTION ( 'NONE',  ( -1.000000000000000000, 0.000000000000000000, 0.000000000000000000 ) ) ;
#13857=CARTESIAN_POINT ( 'NONE',  ( -168.2608473273504615, 32.01710443037316622, 2.601363783521516648 ) ) ;
#13859=EDGE_CURVE ( 'NONE', #1906, #4836, #13192, .T. ) ;
#13867=CARTESIAN_POINT ( 'NONE',  ( -79.20163718375225415, 48.91533818955501545, 2.500000000000000000 ) ) ;
#13875=EDGE_CURVE ( 'NONE', #15554, #16333, #16514, .T. ) ;
#13877=ORIENTED_EDGE ( 'NONE', *, *, #3123, .F. ) ;
#13881=ORIENTED_EDGE ( 'NONE', *, *, #2209, .F. ) ;
#13888=EDGE_CURVE ( 'NONE', #2138, #11597, #16553, .T. ) ;
#13890=DIRECTION ( 'NONE',  ( 0.1856185419698762884, -0.9826218788918641422, 0.000000000000000000 ) ) ;
#13898=VECTOR ( 'NONE', #6501, 1000.000000000000000 ) ;
#13924=ORIENTED_EDGE ( 'NONE', *, *, #16765, .T. ) ;
#13934=AXIS2_PLACEMENT_3D ( 'NONE', #4509, #10292, #8882 ) ;
#13951=VERTEX_POINT ( 'NONE', #7900 ) ;
#13956=CARTESIAN_POINT ( 'NONE',  ( -170.4545578613200121, 32.23085387660965750, -4.766626691765356583 ) ) ;
#13964=CARTESIAN_POINT ( 'NONE',  ( -168.4551535821700838, 31.98984275266787591, 2.662644313562632536 ) ) ;
#13976=AXIS2_PLACEMENT_3D ( 'NONE', #17877, #10354, #417 ) ;
#13996=SURFACE_SIDE_STYLE ('',( #11238 ) ) ;
#14046=ORIENTED_EDGE ( 'NONE', *, *, #8292, .T. ) ;
#14047=ORIENTED_EDGE ( 'NONE', *, *, #13132, .T. ) ;
#14052=CYLINDRICAL_SURFACE ( 'NONE', #2472, 145.0000000000000000 ) ;
#14053=CARTESIAN_POINT ( 'NONE',  ( -169.0003623166909676, 31.93509481583945586, 2.918139657044721336 ) ) ;
#14057=CARTESIAN_POINT ( 'NONE',  ( -70.95370422460223381, 45.40580545587239669, 4.440689772049350559 ) ) ;
#14069=ORIENTED_EDGE ( 'NONE', *, *, #783, .T. ) ;
#14073=VERTEX_POINT ( 'NONE', #16821 ) ;
#14082=FACE_OUTER_BOUND ( 'NONE', #2954, .T. ) ;
#14084=( NAMED_UNIT ( * ) PLANE_ANGLE_UNIT ( ) SI_UNIT ( $, .RADIAN. ) );
#14085=EDGE_CURVE ( 'NONE', #11811, #3590, #5244, .T. ) ;
#14095=CARTESIAN_POINT ( 'NONE',  ( -78.67340168335934436, 1.237153554093905594, 3.655650250101004417 ) ) ;
#14105=CARTESIAN_POINT ( 'NONE',  ( -167.4745151998187680, 32.15905408292206147, -2.500000000000000000 ) ) ;
#14106=EDGE_CURVE ( 'NONE', #14747, #18388, #2290, .T. ) ;
#14112=CARTESIAN_POINT ( 'NONE',  ( -349.6046375497077179, 10.42115585936045896, 9.951701414186830458E-16 ) ) ;
#14130=AXIS2_PLACEMENT_3D ( 'NONE', #3439, #3083, #10464 ) ;
#14157=CARTESIAN_POINT ( 'NONE',  ( -73.57633726875977231, 46.52174766375585335, 2.626980532068773133 ) ) ;
#14167=VERTEX_POINT ( 'NONE', #2359 ) ;
#14182=CYLINDRICAL_SURFACE ( 'NONE', #6789, 2.200000000000000178 ) ;
#14220=EDGE_LOOP ( 'NONE', ( #8267, #3209, #3644, #11867 ) ) ;
#14224=DIRECTION ( 'NONE',  ( -0.1856185419698762329, 0.9826218788918640312, -0.000000000000000000 ) ) ;
#14229=EDGE_LOOP ( 'NONE', ( #7050, #40, #12994, #4686, #15626, #3537, #15148, #12915, #9920, #11419 ) ) ;
#14255=ORIENTED_EDGE ( 'NONE', *, *, #17865, .T. ) ;
#14259=AXIS2_PLACEMENT_3D ( 'NONE', #14920, #2027, #6413 ) ;
#14270=ADVANCED_FACE ( 'NONE', ( #11263 ), #17081, .T. ) ;
#14315=DIRECTION ( 'NONE',  ( 1.000000000000000000, 0.000000000000000000, -0.000000000000000000 ) ) ;
#14316=EDGE_LOOP ( 'NONE', ( #14069, #9337 ) ) ;
#14353=CARTESIAN_POINT ( 'NONE',  ( -76.88766983611584749, -2.536636612185957595, 25.00000000000000000 ) ) ;
#14355=EDGE_CURVE ( 'NONE', #18000, #15303, #13186, .T. ) ;
#14359=CARTESIAN_POINT ( 'NONE',  ( -62.00000000000000000, 0.000000000000000000, 20.00000000000001776 ) ) ;
#14360=CARTESIAN_POINT ( 'NONE',  ( 0.000000000000000000, 0.000000000000000000, -25.00000000000000000 ) ) ;
#14373=EDGE_CURVE ( 'NONE', #17705, #3775, #1615, .T. ) ;
#14377=VECTOR ( 'NONE', #3309, 1000.000000000000227 ) ;
#14387=CARTESIAN_POINT ( 'NONE',  ( -77.60964193335624373, -0.02405657537030136614, 4.939660022666148009 ) ) ;
#14394=VERTEX_POINT ( 'NONE', #5957 ) ;
#14403=AXIS2_PLACEMENT_3D ( 'NONE', #12830, #16846, #12734 ) ;
#14411=EDGE_LOOP ( 'NONE', ( #1624, #10390, #9544, #8791, #4691, #10260 ) ) ;
#14413=ORIENTED_EDGE ( 'NONE', *, *, #7990, .T. ) ;
#14447=CYLINDRICAL_SURFACE ( 'NONE', #6238, 2.200000000000000178 ) ;
#14475=AXIS2_PLACEMENT_3D ( 'NONE', #15860, #288, #6983 ) ;
#14484=FACE_OUTER_BOUND ( 'NONE', #10337, .T. ) ;
#14485=CIRCLE ( 'NONE', #12634, 2.200000000000000178 ) ;
#14513=CARTESIAN_POINT ( 'NONE',  ( -76.98587034812761942, -1.614196834991422858, -6.560995283100326425 ) ) ;
#14544=CARTESIAN_POINT ( 'NONE',  ( -174.0603277000674325, 56.10099541002031742, 3.279750847804461245 ) ) ;
#14547=CARTESIAN_POINT ( 'NONE',  ( -70.11841833929642576, 45.05038753831868803, -6.363771460920504275 ) ) ;
#14554=ORIENTED_EDGE ( 'NONE', *, *, #13342, .T. ) ;
#14575=ORIENTED_EDGE ( 'NONE', *, *, #16610, .T. ) ;
#14576=LINE ( 'NONE', #6236, #15039 ) ;
#14597=LINE ( 'NONE', #10222, #5967 ) ;
#14601=CIRCLE ( 'NONE', #2174, 2.200000000000000178 ) ;
#14606=PLANE ( 'NONE',  #3697 ) ;
#14626=CARTESIAN_POINT ( 'NONE',  ( -175.0988807681447383, 56.35851375132025254, 2.556294622946508611E-15 ) ) ;
#14636=EDGE_CURVE ( 'NONE', #11597, #16602, #6620, .T. ) ;
#14637=CARTESIAN_POINT ( 'NONE',  ( -174.8836357390702005, 55.21905606219750240, -5.316127001577088507 ) ) ;
#14642=AXIS2_PLACEMENT_3D ( 'NONE', #1337, #1515, #17359 ) ;
#14643=LINE ( 'NONE', #6308, #5077 ) ;
#14668=FACE_OUTER_BOUND ( 'NONE', #7621, .T. ) ;
#14676=DIRECTION ( 'NONE',  ( 0.9539392014169441047, 0.3000000000000045963, -2.548423110585629762E-16 ) ) ;
#14690=CARTESIAN_POINT ( 'NONE',  ( -343.6658356661351945, -4.573248343763018475, 9.951701414186830458E-16 ) ) ;
#14694=ORIENTED_EDGE ( 'NONE', *, *, #7223, .F. ) ;
#14697=EDGE_CURVE ( 'NONE', #8575, #8619, #5651, .T. ) ;
#14718=DIRECTION ( 'NONE',  ( 0.000000000000000000, 0.000000000000000000, 1.000000000000000000 ) ) ;
#14739=DIRECTION ( 'NONE',  ( -0.000000000000000000, -0.000000000000000000, -1.000000000000000000 ) ) ;
#14747=VERTEX_POINT ( 'NONE', #4328 ) ;
#14749=ORIENTED_EDGE ( 'NONE', *, *, #13875, .T. ) ;
#14759=DIRECTION ( 'NONE',  ( 1.000000000000000000, 0.000000000000000000, 0.000000000000000000 ) ) ;
#14780=CONICAL_SURFACE ( 'NONE', #13550, 12.74754878398197633, 0.01745329251994333364 ) ;
#14789=DIRECTION ( 'NONE',  ( -1.000000000000000000, 0.000000000000000000, 0.000000000000000000 ) ) ;
#14792=AXIS2_PLACEMENT_3D ( 'NONE', #6059, #16002, #3012 ) ;
#14808=ORIENTED_EDGE ( 'NONE', *, *, #14373, .F. ) ;
#14822=VECTOR ( 'NONE', #16621, 1000.000000000000114 ) ;
#14828=CARTESIAN_POINT ( 'NONE',  ( -81.88695483773778960, -2.621191165925490729, 2.499999999999999112 ) ) ;
#14842=CARTESIAN_POINT ( 'NONE',  ( 73.09088021254186174, 1.387778780781445676E-14, -25.00000000000000000 ) ) ;
#14847=VECTOR ( 'NONE', #7449, 1000.000000000000114 ) ;
#14877=CARTESIAN_POINT ( 'NONE',  ( -349.6046375497077179, 10.42115585936044830, 9.951701414186830458E-16 ) ) ;
#14907=CARTESIAN_POINT ( 'NONE',  ( 0.000000000000000000, 0.000000000000000000, 25.00000000000000000 ) ) ;
#14908=CARTESIAN_POINT ( 'NONE',  ( -74.31765932953604192, 46.83718354949606066, -2.499999999999997780 ) ) ;
#14915=PLANE ( 'NONE',  #7210 ) ;
#14920=CARTESIAN_POINT ( 'NONE',  ( -62.00000000000000000, 0.000000000000000000, -25.00000000000000000 ) ) ;
#14944=DIRECTION ( 'NONE',  ( -0.000000000000000000, -0.000000000000000000, -1.000000000000000000 ) ) ;
#14946=ADVANCED_FACE ( 'NONE', ( #17907 ), #13587, .F. ) ;
#14957=EDGE_CURVE ( 'NONE', #897, #18049, #8984, .T. ) ;
#14958=ORIENTED_EDGE ( 'NONE', *, *, #16094, .F. ) ;
#14967=CARTESIAN_POINT ( 'NONE',  ( -170.5980861165185445, 32.53234180668174247, -5.500000000000001776 ) ) ;
#14972=AXIS2_PLACEMENT_3D ( 'NONE', #1995, #17957, #10701 ) ;
#14979=ORIENTED_EDGE ( 'NONE', *, *, #4950, .F. ) ;
#14983=DIRECTION ( 'NONE',  ( -0.000000000000000000, -0.000000000000000000, 1.000000000000000000 ) ) ;
#15005=CARTESIAN_POINT ( 'NONE',  ( -79.05438463828195950, 1.499069270643396345, 3.389939594122236333 ) ) ;
#15006=CARTESIAN_POINT ( 'NONE',  ( -174.8673125818257006, 55.13264502119463373, -5.500000000000001776 ) ) ;
#15007=CARTESIAN_POINT ( 'NONE',  ( -65.37641414873199608, -43.03264333350146131, -20.00000000000000000 ) ) ;
#15008=AXIS2_PLACEMENT_3D ( 'NONE', #997, #6768, #3878 ) ;
#15023=VERTEX_POINT ( 'NONE', #2132 ) ;
#15034=EDGE_LOOP ( 'NONE', ( #3496, #10126, #2231, #14808, #11475, #6306, #13434, #18614, #7404, #6589 ) ) ;
#15039=VECTOR ( 'NONE', #17723, 1000.000000000000114 ) ;
#15060=EDGE_CURVE ( 'NONE', #16292, #16602, #9730, .T. ) ;
#15068=CYLINDRICAL_SURFACE ( 'NONE', #12535, 171.3327290851023292 ) ;
#15073=EDGE_LOOP ( 'NONE', ( #6475, #3757, #15262, #10601 ) ) ;
#15097=ORIENTED_EDGE ( 'NONE', *, *, #6732, .T. ) ;
#15104=CARTESIAN_POINT ( 'NONE',  ( -173.5975526607244035, 56.27156339024950427, -2.918139657044712454 ) ) ;
#15117=LINE ( 'NONE', #16113, #559 ) ;
#15134=DIRECTION ( 'NONE',  ( 0.000000000000000000, 0.000000000000000000, 1.000000000000000000 ) ) ;
#15144=CARTESIAN_POINT ( 'NONE',  ( -76.88766983611584749, -2.536636612185957595, -7.500000000000000000 ) ) ;
#15148=ORIENTED_EDGE ( 'NONE', *, *, #18484, .F. ) ;
#15200=VERTEX_POINT ( 'NONE', #17219 ) ;
#15205=B_SPLINE_CURVE_WITH_KNOTS ( 'NONE', 3,
 ( #18695, #5667, #16707, #13820, #7289, #16085 ),
 .UNSPECIFIED., .F., .F.,
 ( 4, 2, 4 ),
 ( 0.000000000000000000, 0.001759783889192315272, 0.003519567778384630544 ),
 .UNSPECIFIED. ) ;
#15245=DIRECTION ( 'NONE',  ( -0.9201637183752249260, -0.3915338189555018777, 0.000000000000000000 ) ) ;
#15246=CARTESIAN_POINT ( 'NONE',  ( -169.4331498180839901, 31.75282987493100606, -2.500000000000000000 ) ) ;
#15262=ORIENTED_EDGE ( 'NONE', *, *, #8870, .T. ) ;
#15276=ORIENTED_EDGE ( 'NONE', *, *, #15968, .F. ) ;
#15278=ADVANCED_FACE ( 'NONE', ( #17494 ), #10263, .F. ) ;
#15281=CARTESIAN_POINT ( 'NONE',  ( -170.5817601278045288, 32.44591577653011427, -5.316095106350547717 ) ) ;
#15291=CARTESIAN_POINT ( 'NONE',  ( 73.09088021254186174, 1.387778780781445676E-14, -25.00000000000000000 ) ) ;
#15303=VERTEX_POINT ( 'NONE', #13189 ) ;
#15315=CARTESIAN_POINT ( 'NONE',  ( -176.1167811578620501, -139.6880237571007513, 2.500000000000000000 ) ) ;
#15325=ORIENTED_EDGE ( 'NONE', *, *, #15551, .T. ) ;
#15343=DIRECTION ( 'NONE',  ( 0.9826218788918642533, 0.1856185419698762884, -0.000000000000000000 ) ) ;
#15344=AXIS2_PLACEMENT_3D ( 'NONE', #7018, #12761, #18613 ) ;
#15377=CARTESIAN_POINT ( 'NONE',  ( -170.1316674247146352, 32.02951924490234603, -4.052748550462852428 ) ) ;
#15388=CIRCLE ( 'NONE', #14475, 15.83618137761394173 ) ;
#15417=ADVANCED_FACE ( 'NONE', ( #10904 ), #18271, .F. ) ;
#15419=CARTESIAN_POINT ( 'NONE',  ( -172.7326993491721225, 43.83249341393818810, 5.500000000000000000 ) ) ;
#15426=CARTESIAN_POINT ( 'NONE',  ( 73.09088021254186174, 1.387778780781445676E-14, 25.00000000000000000 ) ) ;
#15428=ORIENTED_EDGE ( 'NONE', *, *, #6296, .F. ) ;
#15431=DIRECTION ( 'NONE',  ( 0.1856185419698762329, -0.9826218788918640312, 0.000000000000000000 ) ) ;
#15434=DIRECTION ( 'NONE',  ( 1.000000000000000000, 0.000000000000000000, -2.631994239413086031E-16 ) ) ;
#15456=EDGE_CURVE ( 'NONE', #3230, #10291, #918, .T. ) ;
#15468=CIRCLE ( 'NONE', #6087, 2.200000000000000178 ) ;
#15474=CARTESIAN_POINT ( 'NONE',  ( 73.09088021254186174, 1.387778780781445676E-14, 7.500000000000000000 ) ) ;
#15494=CARTESIAN_POINT ( 'NONE',  ( -65.23030399291528170, -43.49999999999991473, -19.99999999999999645 ) ) ;
#15495=VECTOR ( 'NONE', #6365, 1000.000000000000000 ) ;
#15514=DIRECTION ( 'NONE',  ( -0.9826218788918642533, -0.1856185419698762884, 0.000000000000000000 ) ) ;
#15523=CARTESIAN_POINT ( 'NONE',  ( -78.35789227062710438, 0.9448366394476784835, 3.952811421308334072 ) ) ;
#15527=DIRECTION ( 'NONE',  ( -1.000000000000000000, 0.000000000000000000, 0.000000000000000000 ) ) ;
#15547=VERTEX_POINT ( 'NONE', #12133 ) ;
#15551=EDGE_CURVE ( 'NONE', #17451, #8575, #10803, .T. ) ;
#15554=VERTEX_POINT ( 'NONE', #8070 ) ;
#15573=CARTESIAN_POINT ( 'NONE',  ( -70.00000000000002842, 45.00000000000000711, 7.169068164496141371 ) ) ;
#15575=CIRCLE ( 'NONE', #14972, 145.0000000000000284 ) ;
#15584=ORIENTED_EDGE ( 'NONE', *, *, #5918, .F. ) ;
#15610=CIRCLE ( 'NONE', #9560, 12.74754878398197633 ) ;
#15611=CARTESIAN_POINT ( 'NONE',  ( -169.4331498180839901, 31.75282987493098474, 2.500000000000000000 ) ) ;
#15612=CARTESIAN_POINT ( 'NONE',  ( -347.2219194661251436, -2.192405777922094678, 9.951701414186830458E-16 ) ) ;
#15620=DIRECTION ( 'NONE',  ( -0.000000000000000000, -0.000000000000000000, -1.000000000000000000 ) ) ;
#15622=DIRECTION ( 'NONE',  ( -1.000000000000000000, 0.000000000000000000, -3.816390434826605238E-17 ) ) ;
#15623=DIRECTION ( 'NONE',  ( 0.1856185419698762329, -0.9826218788918640312, 0.000000000000000000 ) ) ;
#15626=ORIENTED_EDGE ( 'NONE', *, *, #6849, .T. ) ;
#15628=CARTESIAN_POINT ( 'NONE',  ( -62.00000000000000000, 0.000000000000000000, -25.00000000000000000 ) ) ;
#15682=AXIS2_PLACEMENT_3D ( 'NONE', #17702, #3513, #17980 ) ;
#15699=ORIENTED_EDGE ( 'NONE', *, *, #12484, .F. ) ;
#15701=AXIS2_PLACEMENT_3D ( 'NONE', #14359, #16153, #3147 ) ;
#15714=CIRCLE ( 'NONE', #1513, 145.0000000000000284 ) ;
#15728=FACE_OUTER_BOUND ( 'NONE', #9168, .T. ) ;
#15742=CARTESIAN_POINT ( 'NONE',  ( -175.0529311237955596, 56.11526690008648899, 2.500000000000000000 ) ) ;
#15749=CARTESIAN_POINT ( 'NONE',  ( -77.60960976086163043, -0.02410910878642313210, -4.939713573722440465 ) ) ;
#15770=CIRCLE ( 'NONE', #12990, 2.200000000000000178 ) ;
#15798=EDGE_CURVE ( 'NONE', #3590, #15891, #748, .T. ) ;
#15808=ORIENTED_EDGE ( 'NONE', *, *, #7729, .T. ) ;
#15812=ORIENTED_EDGE ( 'NONE', *, *, #10526, .F. ) ;
#15815=CARTESIAN_POINT ( 'NONE',  ( -77.50990852772314099, -0.1964846621953221517, 5.115456906574511464 ) ) ;
#15816=ORIENTED_EDGE ( 'NONE', *, *, #5374, .T. ) ;
#15826=CARTESIAN_POINT ( 'NONE',  ( -79.05438463828194529, 1.499069270643416107, 2.500000000000000000 ) ) ;
#15830=CARTESIAN_POINT ( 'NONE',  ( -74.62210677719829732, 46.96672731380024146, -2.500000000000000000 ) ) ;
#15841=CARTESIAN_POINT ( 'NONE',  ( -77.95461635773787634, 0.4738735750096247923, -4.432276680483205666 ) ) ;
#15849=ORIENTED_EDGE ( 'NONE', *, *, #17409, .T. ) ;
#15850=VERTEX_POINT ( 'NONE', #15144 ) ;
#15860=CARTESIAN_POINT ( 'NONE',  ( -346.6053245638183853, 10.98772995598034008, 9.951701414186830458E-16 ) ) ;
#15868=FACE_OUTER_BOUND ( 'NONE', #17429, .T. ) ;
#15881=DIRECTION ( 'NONE',  ( 0.1856185419698762329, -0.9826218788918640312, 0.000000000000000000 ) ) ;
#15885=ADVANCED_FACE ( 'NONE', ( #11981 ), #2127, .F. ) ;
#15890=CARTESIAN_POINT ( 'NONE',  ( -76.90911978745816668, 1.387778780781445676E-14, 7.500000000000000000 ) ) ;
#15891=VERTEX_POINT ( 'NONE', #9261 ) ;
#15902=LINE ( 'NONE', #15826, #6700 ) ;
#15904=FACE_OUTER_BOUND ( 'NONE', #16954, .T. ) ;
#15951=AXIS2_PLACEMENT_3D ( 'NONE', #6536, #2068, #10689 ) ;
#15968=EDGE_CURVE ( 'NONE', #15547, #13951, #4243, .T. ) ;
#15975=DIRECTION ( 'NONE',  ( -0.9826218788918641422, -0.1856185419698762606, 0.000000000000000000 ) ) ;
#15981=DIRECTION ( 'NONE',  ( 1.000000000000000000, 0.000000000000000000, 0.000000000000000000 ) ) ;
#15998=CIRCLE ( 'NONE', #15682, 2.200000000000000622 ) ;
#16002=DIRECTION ( 'NONE',  ( -0.000000000000000000, -0.000000000000000000, -1.000000000000000000 ) ) ;
#16035=CIRCLE ( 'NONE', #7273, 3.000000000000002665 ) ;
#16040=ORIENTED_EDGE ( 'NONE', *, *, #4626, .T. ) ;
#16046=CYLINDRICAL_SURFACE ( 'NONE', #3662, 2.200000000000000622 ) ;
#16062=CARTESIAN_POINT ( 'NONE',  ( -70.29518329010467426, 45.12560182341311332, -5.734307918512490332 ) ) ;
#16085=CARTESIAN_POINT ( 'NONE',  ( -81.87192997736541145, 3.395211045985502274, 2.500000000000000000 ) ) ;
#16094=EDGE_CURVE ( 'NONE', #15303, #18000, #2147, .T. ) ;
#16113=CARTESIAN_POINT ( 'NONE',  ( 5.481473465377021625, 12.88229205725314763, 25.00000000000000000 ) ) ;
#16130=UNCERTAINTY_MEASURE_WITH_UNIT (LENGTH_MEASURE( 1.000000000000000082E-05 ), #9497, 'distance_accuracy_value', 'NONE');
#16153=DIRECTION ( 'NONE',  ( 2.671473304378624222E-16, 0.000000000000000000, 1.000000000000000000 ) ) ;
#16154=DIRECTION ( 'NONE',  ( 1.000000000000000000, 0.000000000000000000, -2.671473304378624222E-16 ) ) ;
#16206=EDGE_LOOP ( 'NONE', ( #8078, #4451, #2575, #15816, #16524 ) ) ;
#16233=ORIENTED_EDGE ( 'NONE', *, *, #5918, .T. ) ;
#16245=ORIENTED_EDGE ( 'NONE', *, *, #7816, .F. ) ;
#16252=AXIS2_PLACEMENT_3D ( 'NONE', #6434, #6338, #18007 ) ;
#16277=AXIS2_PLACEMENT_3D ( 'NONE', #18536, #4052, #1160 ) ;
#16291=EDGE_CURVE ( 'NONE', #411, #18427, #16377, .T. ) ;
#16292=VERTEX_POINT ( 'NONE', #2232 ) ;
#16296=AXIS2_PLACEMENT_3D ( 'NONE', #8284, #18066, #5143 ) ;
#16328=ORIENTED_EDGE ( 'NONE', *, *, #15060, .F. ) ;
#16333=VERTEX_POINT ( 'NONE', #6797 ) ;
#16352=AXIS2_PLACEMENT_3D ( 'NONE', #2035, #3438, #13585 ) ;
#16354=ORIENTED_EDGE ( 'NONE', *, *, #1331, .T. ) ;
#16361=AXIS2_PLACEMENT_3D ( 'NONE', #5082, #4802, #16680 ) ;
#16377=CIRCLE ( 'NONE', #17917, 150.0000000000000284 ) ;
#16393=CARTESIAN_POINT ( 'NONE',  ( -69.99999999999998579, -45.00000000000000711, 25.00000000000000000 ) ) ;
#16409=CARTESIAN_POINT ( 'NONE',  ( -76.90911978745816668, 1.387778780781445676E-14, 25.00000000000000000 ) ) ;
#16431=VECTOR ( 'NONE', #12871, 1000.000000000000000 ) ;
#16462=PLANE ( 'NONE',  #1679 ) ;
#16476=DIRECTION ( 'NONE',  ( 1.000000000000000000, 0.000000000000000000, 0.000000000000000000 ) ) ;
#16489=DIRECTION ( 'NONE',  ( -0.000000000000000000, -0.000000000000000000, -1.000000000000000000 ) ) ;
#16498=ADVANCED_FACE ( 'NONE', ( #18592 ), #10268, .F. ) ;
#16500=LINE ( 'NONE', #12114, #14377 ) ;
#16514=CIRCLE ( 'NONE', #17134, 13.99999999999999822 ) ;
#16524=ORIENTED_EDGE ( 'NONE', *, *, #11519, .T. ) ;
#16530=CARTESIAN_POINT ( 'NONE',  ( -173.4288256112363342, 56.32277901880416238, -2.821239268406350753 ) ) ;
#16553=B_SPLINE_CURVE_WITH_KNOTS ( 'NONE', 3,
 ( #4308, #10081, #2872, #14547, #8669, #1475, #16062, #1734, #7263, #5840, #3067, #8859, #6007, #11756, #4582, #2113, #6403, #10645, #14908, #17697 ),
 .UNSPECIFIED., .F., .F.,
 ( 4, 2, 2, 2, 2, 2, 2, 2, 2, 4 ),
 ( 0.000000000000000000, 0.0009785969257606898751, 0.001467895388641035463, 0.001957193851521381485, 0.002935790777282072661, 0.003914387703042764705, 0.004892984628803457615, 0.005871581554564148792, 0.006850178480324841702, 0.007828775406085534613 ),
 .UNSPECIFIED. ) ;
#16557=EDGE_CURVE ( 'NONE', #16292, #15023, #4494, .T. ) ;
#16577=DIRECTION ( 'NONE',  ( 1.000000000000000000, 0.000000000000000000, 0.000000000000000000 ) ) ;
#16590=FACE_OUTER_BOUND ( 'NONE', #12409, .T. ) ;
#16602=VERTEX_POINT ( 'NONE', #6114 ) ;
#16605=LINE ( 'NONE', #12416, #4421 ) ;
#16610=EDGE_CURVE ( 'NONE', #56, #14073, #14485, .T. ) ;
#16611=EDGE_LOOP ( 'NONE', ( #2964, #14694, #5524, #6168 ) ) ;
#16621=DIRECTION ( 'NONE',  ( -0.9201637183752250371, 0.3915338189555017112, -0.000000000000000000 ) ) ;
#16635=CARTESIAN_POINT ( 'NONE',  ( -169.4916495677151715, 31.92505963027457483, 3.278196957010509394 ) ) ;
#16653=DIRECTION ( 'NONE',  ( 1.000000000000000000, 0.000000000000000000, -2.671473304378624222E-16 ) ) ;
#16662=VERTEX_POINT ( 'NONE', #512 ) ;
#16680=DIRECTION ( 'NONE',  ( 1.000000000000000000, 0.000000000000000000, 0.000000000000000000 ) ) ;
#16685=PLANE ( 'NONE',  #15951 ) ;
#16687=CIRCLE ( 'NONE', #1855, 2.999999999999999112 ) ;
#16691=CARTESIAN_POINT ( 'NONE',  ( -70.00000000000001421, 44.99999999999998579, 2.500000000000000000 ) ) ;
#16699=EDGE_CURVE ( 'NONE', #7569, #8040, #14643, .T. ) ;
#16700=EDGE_CURVE ( 'NONE', #5412, #4610, #15998, .T. ) ;
#16706=CARTESIAN_POINT ( 'NONE',  ( -172.7326993491721225, 43.83249341393818810, 9.951701414186830458E-16 ) ) ;
#16707=CARTESIAN_POINT ( 'NONE',  ( -79.93235417334217630, 2.099789364928617452, 2.874262317885239781 ) ) ;
#16713=FACE_OUTER_BOUND ( 'NONE', #17402, .T. ) ;
#16721=VERTEX_POINT ( 'NONE', #15005 ) ;
#16736=CARTESIAN_POINT ( 'NONE',  ( -168.8266622669028152, 31.94878367126290897, -2.822349119005427287 ) ) ;
#16744=CARTESIAN_POINT ( 'NONE',  ( -167.4745151998187680, 32.15905408292213252, 2.500000000000000000 ) ) ;
#16759=CARTESIAN_POINT ( 'NONE',  ( -62.00000000000000000, 0.000000000000000000, 25.00000000000000000 ) ) ;
#16761=ORIENTED_EDGE ( 'NONE', *, *, #17993, .T. ) ;
#16765=EDGE_CURVE ( 'NONE', #3705, #10837, #7516, .T. ) ;
#16779=EDGE_LOOP ( 'NONE', ( #7703, #16233 ) ) ;
#16811=EDGE_CURVE ( 'NONE', #11250, #113, #7254, .T. ) ;
#16814=VECTOR ( 'NONE', #9006, 1000.000000000000000 ) ;
#16819=DIRECTION ( 'NONE',  ( 0.000000000000000000, 0.000000000000000000, 1.000000000000000000 ) ) ;
#16821=CARTESIAN_POINT ( 'NONE',  ( 2.200000000000000178, 2.694222958124177006E-16, 25.00000000000000000 ) ) ;
#16841=CARTESIAN_POINT ( 'NONE',  ( -74.31763473078903814, 46.83717308261807943, 2.499999999999997780 ) ) ;
#16846=DIRECTION ( 'NONE',  ( -0.9826218788918642533, -0.1856185419698762884, 0.000000000000000000 ) ) ;
#16849=DIRECTION ( 'NONE',  ( 0.000000000000000000, 0.000000000000000000, 1.000000000000000000 ) ) ;
#16868=ORIENTED_EDGE ( 'NONE', *, *, #2660, .F. ) ;
#16888=CARTESIAN_POINT ( 'NONE',  ( -170.4124675745486570, 31.54971992778987655, -2.500000000000000000 ) ) ;
#16902=ORIENTED_EDGE ( 'NONE', *, *, #14636, .F. ) ;
#16919=VERTEX_POINT ( 'NONE', #17303 ) ;
#16923=CARTESIAN_POINT ( 'NONE',  ( -170.5500457218257679, 32.36841325234162525, -5.132545408516862473 ) ) ;
#16933=CARTESIAN_POINT ( 'NONE',  ( -70.61510477223565374, 45.26172985928680959, 4.986359585138714579 ) ) ;
#16942=ORIENTED_EDGE ( 'NONE', *, *, #10277, .F. ) ;
#16949=PRODUCT_DEFINITION ( 'UNKNOWN', '', #4168, #3390 ) ;
#16954=EDGE_LOOP ( 'NONE', ( #9540, #7318, #10293, #12735, #12877 ) ) ;
#16963=PRESENTATION_STYLE_ASSIGNMENT (( #5074 ) ) ;
#16974=DIRECTION ( 'NONE',  ( -0.000000000000000000, -0.000000000000000000, -1.000000000000000000 ) ) ;
#16983=CARTESIAN_POINT ( 'NONE',  ( -170.5980861165185445, 32.53234180668174247, 5.500000000000001776 ) ) ;
#16988=VECTOR ( 'NONE', #1549, 1000.000000000000000 ) ;
#17008=ORIENTED_EDGE ( 'NONE', *, *, #6638, .F. ) ;
#17042=DIRECTION ( 'NONE',  ( 1.000000000000000000, 0.000000000000000000, 0.000000000000000000 ) ) ;
#17060=DIRECTION ( 'NONE',  ( -0.9201637183752248150, 0.3915338189555022108, 0.000000000000000000 ) ) ;
#17081=CYLINDRICAL_SURFACE ( 'NONE', #1706, 150.0000000000000284 ) ;
#17088=CARTESIAN_POINT ( 'NONE',  ( -172.1050654871199868, 56.67212252599612299, -2.500000000000000000 ) ) ;
#17089=VERTEX_POINT ( 'NONE', #4833 ) ;
#17134=AXIS2_PLACEMENT_3D ( 'NONE', #14360, #14718, #7435 ) ;
#17169=LINE ( 'NONE', #8260, #16431 ) ;
#17192=CIRCLE ( 'NONE', #11403, 150.0000000000000284 ) ;
#17219=CARTESIAN_POINT ( 'NONE',  ( -59.79999999999999716, 0.000000000000000000, -25.00000000000000000 ) ) ;
#17223=PLANE ( 'NONE',  #4405 ) ;
#17258=ORIENTED_EDGE ( 'NONE', *, *, #8750, .F. ) ;
#17277=CARTESIAN_POINT ( 'NONE',  ( -170.3665179301995352, 31.30647307655612366, 9.951701414186830458E-16 ) ) ;
#17279=FACE_BOUND ( 'NONE', #16779, .T. ) ;
#17295=CARTESIAN_POINT ( 'NONE',  ( 5.481473465377026955, -12.88229205725314763, 25.00000000000000000 ) ) ;
#17303=CARTESIAN_POINT ( 'NONE',  ( -71.90911978745813826, 1.387778780781445676E-14, 20.00000000000001421 ) ) ;
#17307=ORIENTED_EDGE ( 'NONE', *, *, #14697, .T. ) ;
#17321=CIRCLE ( 'NONE', #6416, 145.0000000000000284 ) ;
#17325=DIRECTION ( 'NONE',  ( 2.671473304378624222E-16, 0.000000000000000000, 1.000000000000000000 ) ) ;
#17338=CARTESIAN_POINT ( 'NONE',  ( -69.99999999999998579, -45.00000000000000711, -25.00000000000000000 ) ) ;
#17359=DIRECTION ( 'NONE',  ( 1.000000000000000000, 0.000000000000000000, -2.631994239413086031E-16 ) ) ;
#17372=CARTESIAN_POINT ( 'NONE',  ( 5.481473465377021625, 12.88229205725314763, 25.00000000000000000 ) ) ;
#17374=ORIENTED_EDGE ( 'NONE', *, *, #13083, .T. ) ;
#17379=CARTESIAN_POINT ( 'NONE',  ( -174.0670050711101737, 56.28339404658827760, 2.500000000000000000 ) ) ;
#17396=ORIENTED_EDGE ( 'NONE', *, *, #4474, .F. ) ;
#17398=DIRECTION ( 'NONE',  ( -0.000000000000000000, -0.000000000000000000, -1.000000000000000000 ) ) ;
#17400=DIRECTION ( 'NONE',  ( 1.000000000000000000, 0.000000000000000000, 0.000000000000000000 ) ) ;
#17402=EDGE_LOOP ( 'NONE', ( #17307, #8746, #7298, #2097, #15325 ) ) ;
#17409=EDGE_CURVE ( 'NONE', #12460, #5191, #12875, .T. ) ;
#17411=EDGE_LOOP ( 'NONE', ( #15428, #4397, #7071, #13881 ) ) ;
#17423=CARTESIAN_POINT ( 'NONE',  ( -70.00000000000000000, 44.99999999999999289, -19.99999999999998934 ) ) ;
#17429=EDGE_LOOP ( 'NONE', ( #2572, #14255, #1980, #17973 ) ) ;
#17451=VERTEX_POINT ( 'NONE', #17372 ) ;
#17452=DIRECTION ( 'NONE',  ( -0.9201637183752249260, -0.3915338189555018777, -3.511704013281690003E-17 ) ) ;
#17475=EDGE_LOOP ( 'NONE', ( #7699, #8548, #5903, #6514, #11004 ) ) ;
#17490=ADVANCED_FACE ( 'NONE', ( #12683 ), #12585, .F. ) ;
#17494=FACE_OUTER_BOUND ( 'NONE', #2764, .T. ) ;
#17496=CARTESIAN_POINT ( 'NONE',  ( -174.6909448281246569, 55.69916092364878324, -4.223374618371431133 ) ) ;
#17523=CARTESIAN_POINT ( 'NONE',  ( -65.37641414873196766, 43.03264333350143289, -19.99999999999998934 ) ) ;
#17546=EDGE_CURVE ( 'NONE', #16662, #18049, #468, .T. ) ;
#17574=LINE ( 'NONE', #196, #16814 ) ;
#17591=CIRCLE ( 'NONE', #2122, 145.0000000000000284 ) ;
#17603=ORIENTED_EDGE ( 'NONE', *, *, #13859, .F. ) ;
#17615=EDGE_CURVE ( 'NONE', #14073, #18000, #14597, .T. ) ;
#17669=B_SPLINE_CURVE_WITH_KNOTS ( 'NONE', 3,
 ( #7997, #18074, #10815, #13673, #13758, #16530, #15104, #7913, #718, #6498, #12236, #5916, #17496, #4486, #10264, #3066, #14637, #13191 ),
 .UNSPECIFIED., .F., .F.,
 ( 4, 2, 2, 2, 2, 2, 2, 2, 4 ),
 ( 0.000000000000000000, 0.0006036110467293986622, 0.001207222093458797324, 0.001810833140188195661, 0.002414444186917594649, 0.003018055233646993202, 0.003621666280376390455, 0.004225277327105788142, 0.004828888373835185828 ),
 .UNSPECIFIED. ) ;
#17697=CARTESIAN_POINT ( 'NONE',  ( -74.62210677719829732, 46.96672731380024146, -2.500000000000000000 ) ) ;
#17702=CARTESIAN_POINT ( 'NONE',  ( -62.00000000000000000, 0.000000000000000000, 25.00000000000000000 ) ) ;
#17705=VERTEX_POINT ( 'NONE', #3843 ) ;
#17708=CARTESIAN_POINT ( 'NONE',  ( -76.90911978745816668, -45.00000000000000711, 20.00000000000002132 ) ) ;
#17715=EDGE_CURVE ( 'NONE', #15200, #13047, #8084, .T. ) ;
#17723=DIRECTION ( 'NONE',  ( 0.9539392014169441047, 0.3000000000000046518, 0.000000000000000000 ) ) ;
#17735=ADVANCED_FACE ( 'NONE', ( #563 ), #16685, .F. ) ;
#17753=DIRECTION ( 'NONE',  ( 0.1856185419698759831, -0.9826218788918641422, 0.000000000000000000 ) ) ;
#17754=EDGE_CURVE ( 'NONE', #5889, #4539, #12092, .T. ) ;
#17775=EDGE_CURVE ( 'NONE', #16602, #2144, #18431, .T. ) ;
#17780=PLANE ( 'NONE',  #6377 ) ;
#17782=EDGE_CURVE ( 'NONE', #8619, #14167, #17192, .T. ) ;
#17786=ORIENTED_EDGE ( 'NONE', *, *, #14106, .F. ) ;
#17803=EDGE_CURVE ( 'NONE', #11811, #7186, #9587, .T. ) ;
#17820=DIRECTION ( 'NONE',  ( -0.9826218788918642533, -0.1856185419698762884, 0.000000000000000000 ) ) ;
#17835=AXIS2_PLACEMENT_3D ( 'NONE', #13111, #9897, #18764 ) ;
#17856=VECTOR ( 'NONE', #15431, 1000.000000000000227 ) ;
#17865=EDGE_CURVE ( 'NONE', #11250, #6623, #2453, .T. ) ;
#17877=CARTESIAN_POINT ( 'NONE',  ( 73.09088021254186174, 1.387778780781445676E-14, -7.500000000000000000 ) ) ;
#17893=DIRECTION ( 'NONE',  ( 1.000000000000000000, 0.000000000000000000, 0.000000000000000000 ) ) ;
#17898=DIRECTION ( 'NONE',  ( 1.000000000000000000, 0.000000000000000000, 0.000000000000000000 ) ) ;
#17907=FACE_OUTER_BOUND ( 'NONE', #12832, .T. ) ;
#17917=AXIS2_PLACEMENT_3D ( 'NONE', #14842, #1863, #5060 ) ;
#17950=FACE_OUTER_BOUND ( 'NONE', #13778, .T. ) ;
#17952=CARTESIAN_POINT ( 'NONE',  ( 5.481473465377021625, 12.88229205725314763, 25.00000000000000000 ) ) ;
#17954=AXIS2_PLACEMENT_3D ( 'NONE', #16706, #2268, #6651 ) ;
#17957=DIRECTION ( 'NONE',  ( -2.671473304378624222E-16, -0.000000000000000000, -1.000000000000000000 ) ) ;
#17971=ORIENTED_EDGE ( 'NONE', *, *, #14106, .T. ) ;
#17973=ORIENTED_EDGE ( 'NONE', *, *, #8979, .F. ) ;
#17980=DIRECTION ( 'NONE',  ( 1.000000000000000000, 0.000000000000000000, 0.000000000000000000 ) ) ;
#17985=ORIENTED_EDGE ( 'NONE', *, *, #2903, .F. ) ;
#17991=ADVANCED_FACE ( 'NONE', ( #10548 ), #14915, .F. ) ;
#17993=EDGE_CURVE ( 'NONE', #3138, #14747, #1162, .T. ) ;
#18000=VERTEX_POINT ( 'NONE', #13391 ) ;
#18007=DIRECTION ( 'NONE',  ( -1.000000000000000000, 0.000000000000000000, 0.000000000000000000 ) ) ;
#18014=DIRECTION ( 'NONE',  ( 0.1856185419698760941, -0.9826218788918640312, 0.000000000000000000 ) ) ;
#18049=VERTEX_POINT ( 'NONE', #15007 ) ;
#18056=ORIENTED_EDGE ( 'NONE', *, *, #564, .T. ) ;
#18066=DIRECTION ( 'NONE',  ( 2.671473304378624222E-16, 0.000000000000000000, 1.000000000000000000 ) ) ;
#18074=CARTESIAN_POINT ( 'NONE',  ( -172.2963380567813942, 56.58533696229243048, -2.499999999999999556 ) ) ;
#18079=CARTESIAN_POINT ( 'NONE',  ( -59.79999999999999716, 0.000000000000000000, 25.00000000000000000 ) ) ;
#18084=DIRECTION ( 'NONE',  ( -0.000000000000000000, -0.000000000000000000, -1.000000000000000000 ) ) ;
#18106=FILL_AREA_STYLE ('',( #8022 ) ) ;
#18122=ORIENTED_EDGE ( 'NONE', *, *, #5318, .F. ) ;
#18126=FACE_OUTER_BOUND ( 'NONE', #7001, .T. ) ;
#18133=CARTESIAN_POINT ( 'NONE',  ( -79.94364498743971126, 2.107449674570485154, -2.869442248077125779 ) ) ;
#18148=ORIENTED_EDGE ( 'NONE', *, *, #11094, .F. ) ;
#18150=DIRECTION ( 'NONE',  ( 0.000000000000000000, 0.000000000000000000, 1.000000000000000000 ) ) ;
#18155=( GEOMETRIC_REPRESENTATION_CONTEXT ( 3 ) GLOBAL_UNCERTAINTY_ASSIGNED_CONTEXT ( ( #6981 ) ) GLOBAL_UNIT_ASSIGNED_CONTEXT ( ( #18508, #14084, #7943 ) ) REPRESENTATION_CONTEXT ( 'NONE', 'WORKASPACE' ) );
#18192=EDGE_CURVE ( 'NONE', #10083, #10544, #2787, .T. ) ;
#18217=CARTESIAN_POINT ( 'NONE',  ( 73.09088021254186174, 1.387778780781445676E-14, 7.500000000000000000 ) ) ;
#18228=CARTESIAN_POINT ( 'NONE',  ( -136.4286012789710867, -132.1908753210555574, 2.500000000000000000 ) ) ;
#18231=CARTESIAN_POINT ( 'NONE',  ( 73.09088021254186174, 1.387778780781445676E-14, 19.99999999999997513 ) ) ;
#18236=CARTESIAN_POINT ( 'NONE',  ( -64.20000000000000284, 2.694222958124175527E-16, -20.00000000000000000 ) ) ;
#18237=VECTOR ( 'NONE', #9905, 1000.000000000000000 ) ;
#18244=CARTESIAN_POINT ( 'NONE',  ( -79.05438463828195950, 1.499069270643396345, -3.389939594122236333 ) ) ;
#18248=DIRECTION ( 'NONE',  ( -0.9826218788918642533, -0.1856185419698762884, 0.000000000000000000 ) ) ;
#18271=PLANE ( 'NONE',  #289 ) ;
#18273=CARTESIAN_POINT ( 'NONE',  ( -70.00000000000000000, 44.99999999999999289, 20.00000000000002132 ) ) ;
#18285=CARTESIAN_POINT ( 'NONE',  ( -169.7748756787665059, 31.94743695617602341, 3.563338245596213039 ) ) ;
#18286=STYLED_ITEM ( 'NONE', ( #12311 ), #8769 ) ;
#18290=CARTESIAN_POINT ( 'NONE',  ( -72.31226064957499489, 45.98387735189907488, 3.156966122918108741 ) ) ;
#18302=ORIENTED_EDGE ( 'NONE', *, *, #6271, .T. ) ;
#18312=FACE_OUTER_BOUND ( 'NONE', #6288, .T. ) ;
#18335=DIRECTION ( 'NONE',  ( -0.000000000000000000, -0.000000000000000000, -1.000000000000000000 ) ) ;
#18358=EDGE_CURVE ( 'NONE', #17451, #13951, #395, .T. ) ;
#18365=CARTESIAN_POINT ( 'NONE',  ( 0.000000000000000000, 0.000000000000000000, -19.99999999999999645 ) ) ;
#18367=CARTESIAN_POINT ( 'NONE',  ( -169.4934689854139549, 31.92509550690243003, -3.279750847804471903 ) ) ;
#18374=CARTESIAN_POINT ( 'NONE',  ( -170.2272147085104166, 32.06920008862883975, 4.223374618371441791 ) ) ;
#18388=VERTEX_POINT ( 'NONE', #679 ) ;
#18397=EDGE_LOOP ( 'NONE', ( #4834, #5758, #6647, #6660 ) ) ;
#18405=( NAMED_UNIT ( * ) SI_UNIT ( $, .STERADIAN. ) SOLID_ANGLE_UNIT ( ) );
#18408=EDGE_CURVE ( 'NONE', #11722, #6775, #11349, .T. ) ;
#18418=CARTESIAN_POINT ( 'NONE',  ( 0.000000000000000000, 0.000000000000000000, 20.00000000000000000 ) ) ;
#18423=CIRCLE ( 'NONE', #860, 171.3327290851023292 ) ;
#18427=VERTEX_POINT ( 'NONE', #3956 ) ;
#18428=ORIENTED_EDGE ( 'NONE', *, *, #16700, .F. ) ;
#18429=AXIS2_PLACEMENT_3D ( 'NONE', #8877, #14739, #6031 ) ;
#18430=CARTESIAN_POINT ( 'NONE',  ( -2.200000000000000178, 0.000000000000000000, 25.00000000000000000 ) ) ;
#18431=CIRCLE ( 'NONE', #4139, 149.4844750268701148 ) ;
#18446=DIRECTION ( 'NONE',  ( 1.000000000000000000, 0.000000000000000000, 0.000000000000000000 ) ) ;
#18472=CARTESIAN_POINT ( 'NONE',  ( 73.09088021254186174, 1.387778780781445676E-14, -19.99999999999999645 ) ) ;
#18479=CARTESIAN_POINT ( 'NONE',  ( -351.9873556332902922, 23.03471749664299395, 2.567204941047428095E-15 ) ) ;
#18484=EDGE_CURVE ( 'NONE', #5191, #10544, #11587, .T. ) ;
#18488=ORIENTED_EDGE ( 'NONE', *, *, #4266, .F. ) ;
#18508=( LENGTH_UNIT ( ) NAMED_UNIT ( * ) SI_UNIT ( .MILLI., .METRE. ) );
#18528=EDGE_CURVE ( 'NONE', #8040, #3775, #8420, .T. ) ;
#18536=CARTESIAN_POINT ( 'NONE',  ( -62.00000000000000000, 0.000000000000000000, -25.00000000000000000 ) ) ;
#18543=PRODUCT ( 'Upper Squeezer Handle Arm', 'Upper Squeezer Handle Arm', '', ( #18667 ) ) ;
#18555=DIRECTION ( 'NONE',  ( 0.1856185419698762329, -0.9826218788918640312, 0.000000000000000000 ) ) ;
#18575=CARTESIAN_POINT ( 'NONE',  ( -70.00000000000000000, 44.99999999999999289, -25.00000000000000000 ) ) ;
#18580=LINE ( 'NONE', #14353, #883 ) ;
#18592=FACE_OUTER_BOUND ( 'NONE', #18397, .T. ) ;
#18598=ADVANCED_FACE ( 'NONE', ( #15904 ), #2744, .F. ) ;
#18599=CARTESIAN_POINT ( 'NONE',  ( -70.00000000000000000, 44.99999999999999289, 25.00000000000000000 ) ) ;
#18613=DIRECTION ( 'NONE',  ( -1.000000000000000000, 0.000000000000000000, 0.000000000000000000 ) ) ;
#18614=ORIENTED_EDGE ( 'NONE', *, *, #12195, .T. ) ;
#18616=CARTESIAN_POINT ( 'NONE',  ( -79.05438463828195950, 1.499069270643396345, 3.389939594122236333 ) ) ;
#18635=AXIS2_PLACEMENT_3D ( 'NONE', #7120, #88, #10204 ) ;
#18653=DIRECTION ( 'NONE',  ( -0.9826218788918640312, -0.1856185419698769823, 0.000000000000000000 ) ) ;
#18664=CARTESIAN_POINT ( 'NONE',  ( -170.5980861165185445, 32.53234180668174247, 5.500000000000001776 ) ) ;
#18667=PRODUCT_CONTEXT ( 'NONE', #5926, 'mechanical' ) ;
#18686=LINE ( 'NONE', #11408, #7604 ) ;
#18695=CARTESIAN_POINT ( 'NONE',  ( -79.05438463828195950, 1.499069270643396345, 3.389939594122236333 ) ) ;
#18712=VECTOR ( 'NONE', #17060, 1000.000000000000000 ) ;
#18741=ORIENTED_EDGE ( 'NONE', *, *, #12741, .F. ) ;
#18747=PLANE ( 'NONE',  #9137 ) ;
#18752=ADVANCED_FACE ( 'NONE', ( #6057 ), #14780, .T. ) ;
#18755=SHAPE_DEFINITION_REPRESENTATION ( #10586, #5397 ) ;
#18763=ORIENTED_EDGE ( 'NONE', *, *, #2209, .T. ) ;
#18764=DIRECTION ( 'NONE',  ( 1.000000000000000000, 0.000000000000000000, 0.000000000000000000 ) ) ;
#18772=AXIS2_PLACEMENT_3D ( 'NONE', #13611, #7473, #14759 ) ;
#18776=CLOSED_SHELL ( 'NONE', ( #17490, #7583, #9445, #18752, #6197, #3988, #9617, #14270, #9348, #11409, #12640, #13770, #17735, #11330, #10080, #9244, #6557, #16498, #1527, #13594, #12769, #7422, #7545, #18598, #5695, #2172, #14946, #10964, #2691, #13021, #15417, #552, #1220, #8864, #9584, #15885, #7329, #7890, #13458, #17991, #2574, #5324, #4515, #11386, #15278, #2687, #4811, #9469 ) ) ;
ENDSEC;
END-ISO-10303-21;
